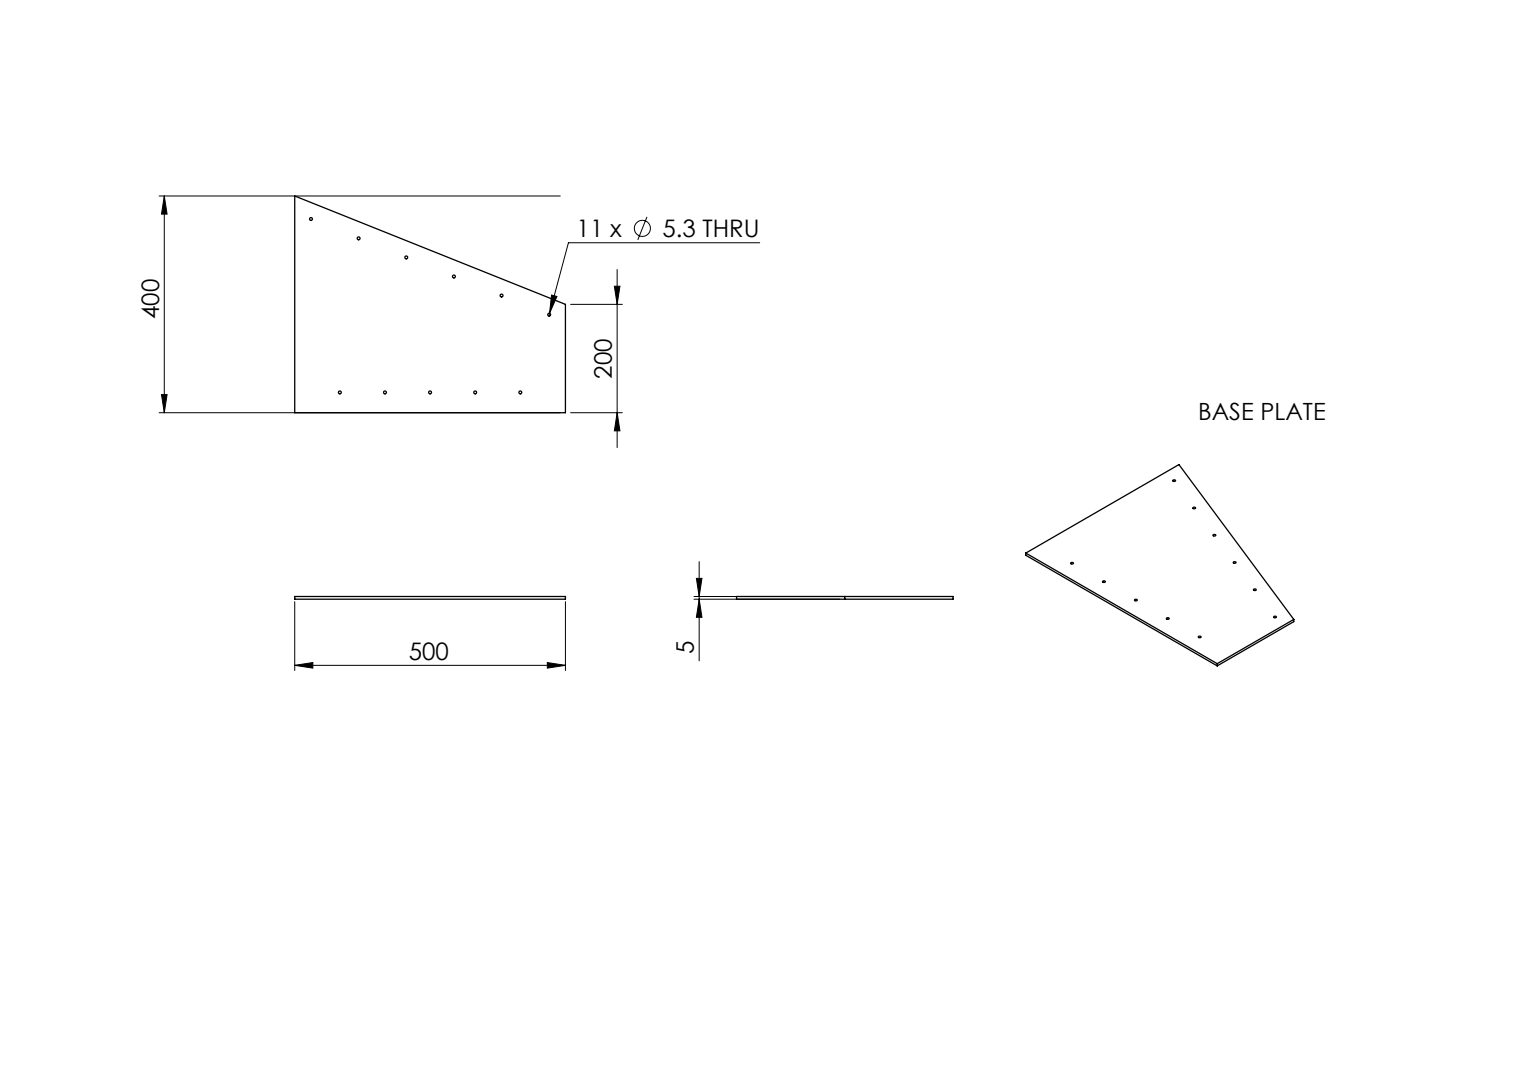
ISO-10303-21;
HEADER;
FILE_DESCRIPTION (('STEP AP214'),
    '1' );
FILE_NAME ('base plate.step',
    '2026-10-24T11:01:53',
    ( '' ),
    ( '' ),
    'SwSTEP 2.0',
    'SolidWorks 2026',
    '' );
FILE_SCHEMA (( 'AUTOMOTIVE_DESIGN' ));
ENDSEC;

DATA;
#2=DIRECTION ( 'NONE',  ( 0.000000000000000000, 0.000000000000000000, 1.000000000000000000 ) ) ;
#30=EDGE_CURVE ( 'NONE', #66, #5441, #6753, .T. ) ;
#34=CIRCLE ( 'NONE', #8257, 2.649999999999985700 ) ;
#39=CARTESIAN_POINT ( 'NONE',  ( 264.0000000000000000, -20.00000000000000000, -48.78142504031547588 ) ) ;
#45=CARTESIAN_POINT ( 'NONE',  ( 352.0000000000000000, -25.00000000000000000, -18.88142504031545243 ) ) ;
#50=DIRECTION ( 'NONE',  ( -0.000000000000000000, 1.000000000000000000, -0.000000000000000000 ) ) ;
#66=VERTEX_POINT ( 'NONE', #8006 ) ;
#72=DIRECTION ( 'NONE',  ( 0.000000000000000000, 0.000000000000000000, 1.000000000000000000 ) ) ;
#74=EDGE_LOOP ( 'NONE', ( #3526, #1411, #5391, #5718 ) ) ;
#79=DIRECTION ( 'NONE',  ( 0.000000000000000000, 0.000000000000000000, 1.000000000000000000 ) ) ;
#80=CIRCLE ( 'NONE', #1767, 2.649999999999985700 ) ;
#95=ORIENTED_EDGE ( 'NONE', *, *, #1233, .T. ) ;
#99=EDGE_LOOP ( 'NONE', ( #6356, #2611 ) ) ;
#101=VERTEX_POINT ( 'NONE', #4083 ) ;
#106=ORIENTED_EDGE ( 'NONE', *, *, #3433, .T. ) ;
#108=CIRCLE ( 'NONE', #2620, 2.649999999999985700 ) ;
#116=LINE ( 'NONE', #6740, #7265 ) ;
#151=CARTESIAN_POINT ( 'NONE',  ( 264.0000000000000000, -20.00000000000000000, -51.43142504031546025 ) ) ;
#152=CARTESIAN_POINT ( 'NONE',  ( 0.000000000000000000, -20.00000000000000000, -154.8500000000000512 ) ) ;
#171=VECTOR ( 'NONE', #2949, 1000.000000000000000 ) ;
#173=VECTOR ( 'NONE', #7716, 1000.000000000000000 ) ;
#196=AXIS2_PLACEMENT_3D ( 'NONE', #7241, #2034, #5327 ) ;
#213=AXIS2_PLACEMENT_3D ( 'NONE', #3905, #5378, #2079 ) ;
#219=CARTESIAN_POINT ( 'NONE',  ( 386.6666666666666288, -20.00000000000000000, 162.5000000000000853 ) ) ;
#228=ORIENTED_EDGE ( 'NONE', *, *, #2374, .T. ) ;
#229=ORIENTED_EDGE ( 'NONE', *, *, #1735, .F. ) ;
#235=EDGE_CURVE ( 'NONE', #6809, #4852, #8223, .T. ) ;
#246=DIRECTION ( 'NONE',  ( 0.000000000000000000, 1.000000000000000000, 0.000000000000000000 ) ) ;
#257=AXIS2_PLACEMENT_3D ( 'NONE', #4957, #2556, #3896 ) ;
#288=EDGE_CURVE ( 'NONE', #3976, #6369, #1904, .T. ) ;
#292=ORIENTED_EDGE ( 'NONE', *, *, #6462, .T. ) ;
#295=EDGE_LOOP ( 'NONE', ( #7507, #2657, #3424, #1885 ) ) ;
#301=AXIS2_PLACEMENT_3D ( 'NONE', #6411, #4498, #8473 ) ;
#359=CIRCLE ( 'NONE', #3284, 2.649999999999985700 ) ;
#372=SURFACE_STYLE_USAGE ( .BOTH. , #1644 ) ;
#376=ORIENTED_EDGE ( 'NONE', *, *, #8589, .T. ) ;
#382=EDGE_LOOP ( 'NONE', ( #940, #229 ) ) ;
#387=LINE ( 'NONE', #1178, #6990 ) ;
#397=ADVANCED_FACE ( 'NONE', ( #5238 ), #7161, .F. ) ;
#402=PLANE ( 'NONE',  #6759 ) ;
#414=DIRECTION ( 'NONE',  ( -0.000000000000000000, 1.000000000000000000, -0.000000000000000000 ) ) ;
#417=CARTESIAN_POINT ( 'NONE',  ( 0.000000000000000000, -20.00000000000000000, -157.5000000000000284 ) ) ;
#424=PRODUCT_DEFINITION ( 'UNKNOWN', '', #7110, #637 ) ;
#437=VERTEX_POINT ( 'NONE', #5072 ) ;
#439=ADVANCED_FACE ( 'NONE', ( #6505 ), #3771, .T. ) ;
#449=VECTOR ( 'NONE', #5880, 1000.000000000000000 ) ;
#452=DIRECTION ( 'NONE',  ( 0.000000000000000000, 0.000000000000000000, 1.000000000000000000 ) ) ;
#453=AXIS2_PLACEMENT_3D ( 'NONE', #5882, #3158, #8554 ) ;
#461=DIRECTION ( 'NONE',  ( 0.000000000000000000, 1.000000000000000000, 0.000000000000000000 ) ) ;
#462=COLOUR_RGB ( '',0.8941176470588234615, 0.8941176470588234615, 0.8941176470588234615 ) ;
#463=ORIENTED_EDGE ( 'NONE', *, *, #2493, .F. ) ;
#464=DIRECTION ( 'NONE',  ( 0.000000000000000000, 0.000000000000000000, 1.000000000000000000 ) ) ;
#469=CIRCLE ( 'NONE', #5320, 2.649999999999985700 ) ;
#487=ORIENTED_EDGE ( 'NONE', *, *, #5222, .T. ) ;
#492=FACE_BOUND ( 'NONE', #3080, .T. ) ;
#499=VECTOR ( 'NONE', #1824, 1000.000000000000000 ) ;
#511=AXIS2_PLACEMENT_3D ( 'NONE', #6789, #836, #2326 ) ;
#523=DIRECTION ( 'NONE',  ( -0.000000000000000000, -0.000000000000000000, -1.000000000000000000 ) ) ;
#532=FACE_BOUND ( 'NONE', #1186, .T. ) ;
#534=DIRECTION ( 'NONE',  ( 0.000000000000000000, 1.000000000000000000, 0.000000000000000000 ) ) ;
#541=CARTESIAN_POINT ( 'NONE',  ( 136.6666666666666288, -20.00000000000000000, 159.8500000000001080 ) ) ;
#542=VERTEX_POINT ( 'NONE', #2423 ) ;
#557=ADVANCED_FACE ( 'NONE', ( #3066, #4491, #7149, #1189, #3755, #5751, #532, #2545, #5707, #1264, #492, #1890 ), #402, .F. ) ;
#558=ORIENTED_EDGE ( 'NONE', *, *, #1197, .T. ) ;
#583=CARTESIAN_POINT ( 'NONE',  ( 219.9999999999999716, -20.00000000000000000, 162.5000000000000853 ) ) ;
#587=AXIS2_PLACEMENT_3D ( 'NONE', #8475, #2553, #2629 ) ;
#590=VERTEX_POINT ( 'NONE', #1227 ) ;
#594=AXIS2_PLACEMENT_3D ( 'NONE', #3123, #464, #5764 ) ;
#602=ORIENTED_EDGE ( 'NONE', *, *, #5769, .F. ) ;
#626=DIRECTION ( 'NONE',  ( 0.000000000000000000, 0.000000000000000000, 1.000000000000000000 ) ) ;
#627=EDGE_CURVE ( 'NONE', #5001, #8500, #3020, .T. ) ;
#635=CARTESIAN_POINT ( 'NONE',  ( 88.00000000000000000, -20.00000000000000000, -121.8314250403154659 ) ) ;
#637=PRODUCT_DEFINITION_CONTEXT ( 'detailed design', #7921, 'design' ) ;
#645=ORIENTED_EDGE ( 'NONE', *, *, #8589, .F. ) ;
#678=VERTEX_POINT ( 'NONE', #39 ) ;
#699=DIRECTION ( 'NONE',  ( 0.000000000000000000, 0.000000000000000000, 1.000000000000000000 ) ) ;
#701=LINE ( 'NONE', #6002, #1786 ) ;
#702=VERTEX_POINT ( 'NONE', #1004 ) ;
#713=ORIENTED_EDGE ( 'NONE', *, *, #3006, .F. ) ;
#723=PLANE ( 'NONE',  #213 ) ;
#742=ADVANCED_FACE ( 'NONE', ( #3927 ), #2016, .F. ) ;
#745=EDGE_CURVE ( 'NONE', #1823, #8068, #1628, .T. ) ;
#769=CARTESIAN_POINT ( 'NONE',  ( 88.00000000000000000, -20.00000000000000000, -119.1814250403154745 ) ) ;
#770=FACE_OUTER_BOUND ( 'NONE', #6133, .T. ) ;
#790=ORIENTED_EDGE ( 'NONE', *, *, #3133, .F. ) ;
#794=EDGE_CURVE ( 'NONE', #7699, #1878, #8026, .T. ) ;
#807=VERTEX_POINT ( 'NONE', #1006 ) ;
#811=EDGE_LOOP ( 'NONE', ( #463, #5711, #6252, #6400 ) ) ;
#818=EDGE_LOOP ( 'NONE', ( #7207, #3911, #376, #7380 ) ) ;
#821=CIRCLE ( 'NONE', #5944, 2.649999999999985700 ) ;
#825=DIRECTION ( 'NONE',  ( -0.000000000000000000, 1.000000000000000000, -0.000000000000000000 ) ) ;
#835=AXIS2_PLACEMENT_3D ( 'NONE', #4055, #2668, #1934 ) ;
#836=DIRECTION ( 'NONE',  ( -0.000000000000000000, 1.000000000000000000, -0.000000000000000000 ) ) ;
#843=DIRECTION ( 'NONE',  ( -0.000000000000000000, -0.000000000000000000, -1.000000000000000000 ) ) ;
#851=EDGE_LOOP ( 'NONE', ( #4373, #2830 ) ) ;
#871=AXIS2_PLACEMENT_3D ( 'NONE', #6654, #7187, #699 ) ;
#873=DIRECTION ( 'NONE',  ( -0.000000000000000000, 1.000000000000000000, -0.000000000000000000 ) ) ;
#875=ORIENTED_EDGE ( 'NONE', *, *, #2374, .F. ) ;
#878=FACE_BOUND ( 'NONE', #2157, .T. ) ;
#912=DIRECTION ( 'NONE',  ( -0.000000000000000000, 1.000000000000000000, -0.000000000000000000 ) ) ;
#921=FACE_BOUND ( 'NONE', #2013, .T. ) ;
#929=AXIS2_PLACEMENT_3D ( 'NONE', #4850, #7548, #4148 ) ;
#937=AXIS2_PLACEMENT_3D ( 'NONE', #5438, #5912, #7446 ) ;
#940=ORIENTED_EDGE ( 'NONE', *, *, #2023, .F. ) ;
#952=EDGE_LOOP ( 'NONE', ( #6894, #7607 ) ) ;
#965=CARTESIAN_POINT ( 'NONE',  ( -30.00000000000002842, -20.00000000000000000, 200.0000000000000000 ) ) ;
#969=ORIENTED_EDGE ( 'NONE', *, *, #7360, .F. ) ;
#995=CARTESIAN_POINT ( 'NONE',  ( 88.00000000000000000, -20.00000000000000000, -121.8314250403154659 ) ) ;
#996=DIRECTION ( 'NONE',  ( 0.000000000000000000, 1.000000000000000000, 0.000000000000000000 ) ) ;
#997=VERTEX_POINT ( 'NONE', #1752 ) ;
#1000=ORIENTED_EDGE ( 'NONE', *, *, #1573, .F. ) ;
#1004=CARTESIAN_POINT ( 'NONE',  ( 0.000000000000000000, -25.00000000000000000, -154.8500000000000512 ) ) ;
#1006=CARTESIAN_POINT ( 'NONE',  ( 264.0000000000000000, -20.00000000000000000, -54.08142504031544462 ) ) ;
#1019=VECTOR ( 'NONE', #8238, 1000.000000000000000 ) ;
#1031=EDGE_LOOP ( 'NONE', ( #8342, #5767, #3173, #2916 ) ) ;
#1058=ADVANCED_FACE ( 'NONE', ( #8581 ), #3438, .F. ) ;
#1060=CARTESIAN_POINT ( 'NONE',  ( 470.0000000000000000, -20.00000000000000000, 200.0000000000000000 ) ) ;
#1077=VERTEX_POINT ( 'NONE', #6603 ) ;
#1100=ORIENTED_EDGE ( 'NONE', *, *, #2407, .F. ) ;
#1112=DIRECTION ( 'NONE',  ( 0.000000000000000000, 0.000000000000000000, 1.000000000000000000 ) ) ;
#1124=CARTESIAN_POINT ( 'NONE',  ( 219.9999999999999716, -20.00000000000000000, 159.8500000000001080 ) ) ;
#1132=ORIENTED_EDGE ( 'NONE', *, *, #1493, .F. ) ;
#1134=LINE ( 'NONE', #5133, #3405 ) ;
#1160=VERTEX_POINT ( 'NONE', #4912 ) ;
#1168=EDGE_CURVE ( 'NONE', #8068, #1823, #2321, .T. ) ;
#1169=ADVANCED_FACE ( 'NONE', ( #2314 ), #6779, .F. ) ;
#1171=ORIENTED_EDGE ( 'NONE', *, *, #5798, .F. ) ;
#1174=CARTESIAN_POINT ( 'NONE',  ( 219.9999999999999716, -20.00000000000000000, 162.5000000000000853 ) ) ;
#1178=CARTESIAN_POINT ( 'NONE',  ( 219.9999999999999716, -20.00000000000000000, 165.1500000000000625 ) ) ;
#1186=EDGE_LOOP ( 'NONE', ( #3554, #4363 ) ) ;
#1189=FACE_BOUND ( 'NONE', #5501, .T. ) ;
#1190=DIRECTION ( 'NONE',  ( 0.000000000000000000, 0.000000000000000000, 1.000000000000000000 ) ) ;
#1197=EDGE_CURVE ( 'NONE', #4852, #5678, #6117, .T. ) ;
#1202=CYLINDRICAL_SURFACE ( 'NONE', #4532, 2.649999999999985700 ) ;
#1207=LINE ( 'NONE', #3864, #3823 ) ;
#1219=CARTESIAN_POINT ( 'NONE',  ( 88.00000000000000000, -25.00000000000000000, -119.1814250403154745 ) ) ;
#1226=EDGE_CURVE ( 'NONE', #702, #8500, #2952, .T. ) ;
#1227=CARTESIAN_POINT ( 'NONE',  ( 303.3333333333333144, -20.00000000000000000, 165.1500000000000625 ) ) ;
#1233=EDGE_CURVE ( 'NONE', #5259, #66, #3566, .T. ) ;
#1264=FACE_BOUND ( 'NONE', #2961, .T. ) ;
#1283=ORIENTED_EDGE ( 'NONE', *, *, #5388, .F. ) ;
#1285=AXIS2_PLACEMENT_3D ( 'NONE', #7939, #6622, #1975 ) ;
#1292=CARTESIAN_POINT ( 'NONE',  ( 219.9999999999999716, -20.00000000000000000, 162.5000000000000853 ) ) ;
#1311=LINE ( 'NONE', #7982, #7625 ) ;
#1325=EDGE_LOOP ( 'NONE', ( #7906, #6774 ) ) ;
#1336=ORIENTED_EDGE ( 'NONE', *, *, #1493, .T. ) ;
#1339=AXIS2_PLACEMENT_3D ( 'NONE', #5714, #7733, #452 ) ;
#1344=AXIS2_PLACEMENT_3D ( 'NONE', #2621, #6085, #6001 ) ;
#1346=CARTESIAN_POINT ( 'NONE',  ( 352.0000000000000000, -20.00000000000000000, -16.23142504031546807 ) ) ;
#1364=CIRCLE ( 'NONE', #3460, 2.649999999999985700 ) ;
#1369=UNCERTAINTY_MEASURE_WITH_UNIT (LENGTH_MEASURE( 1.000000000000000082E-05 ), #4293, 'distance_accuracy_value', 'NONE');
#1370=ORIENTED_EDGE ( 'NONE', *, *, #1684, .T. ) ;
#1371=DIRECTION ( 'NONE',  ( 0.000000000000000000, 0.000000000000000000, 1.000000000000000000 ) ) ;
#1376=EDGE_LOOP ( 'NONE', ( #713, #2858, #5114, #8177 ) ) ;
#1385=ORIENTED_EDGE ( 'NONE', *, *, #1994, .T. ) ;
#1388=CARTESIAN_POINT ( 'NONE',  ( 352.0000000000000000, -25.00000000000000000, -13.58142504031548192 ) ) ;
#1404=CARTESIAN_POINT ( 'NONE',  ( 352.0000000000000000, -20.00000000000000000, -16.23142504031546807 ) ) ;
#1409=EDGE_LOOP ( 'NONE', ( #2213, #1591 ) ) ;
#1411=ORIENTED_EDGE ( 'NONE', *, *, #8314, .T. ) ;
#1412=EDGE_LOOP ( 'NONE', ( #1000, #1132, #7088, #5511 ) ) ;
#1429=ADVANCED_FACE ( 'NONE', ( #8407 ), #2446, .F. ) ;
#1431=DIRECTION ( 'NONE',  ( -0.000000000000000000, 1.000000000000000000, -0.000000000000000000 ) ) ;
#1450=FACE_OUTER_BOUND ( 'NONE', #2004, .T. ) ;
#1451=CARTESIAN_POINT ( 'NONE',  ( 136.6666666666666288, -20.00000000000000000, 165.1500000000000625 ) ) ;
#1458=CARTESIAN_POINT ( 'NONE',  ( 439.9999999999999432, -20.00000000000000000, 18.96857495968446017 ) ) ;
#1462=CARTESIAN_POINT ( 'NONE',  ( 53.33333333333330017, -25.00000000000000000, 165.1500000000000625 ) ) ;
#1469=LINE ( 'NONE', #8144, #2419 ) ;
#1471=AXIS2_PLACEMENT_3D ( 'NONE', #2548, #5905, #72 ) ;
#1493=EDGE_CURVE ( 'NONE', #1660, #542, #6479, .T. ) ;
#1499=DIRECTION ( 'NONE',  ( 0.000000000000000000, 1.000000000000000000, 0.000000000000000000 ) ) ;
#1512=PRODUCT_CONTEXT ( 'NONE', #2313, 'mechanical' ) ;
#1528=DIRECTION ( 'NONE',  ( 0.000000000000000000, -0.000000000000000000, 1.000000000000000000 ) ) ;
#1540=CARTESIAN_POINT ( 'NONE',  ( 53.33333333333330017, -20.00000000000000000, 159.8500000000001080 ) ) ;
#1570=ADVANCED_FACE ( 'NONE', ( #6676 ), #723, .F. ) ;
#1573=EDGE_CURVE ( 'NONE', #542, #807, #4727, .T. ) ;
#1577=VECTOR ( 'NONE', #6770, 1000.000000000000000 ) ;
#1591=ORIENTED_EDGE ( 'NONE', *, *, #7360, .T. ) ;
#1593=EDGE_CURVE ( 'NONE', #4392, #5678, #6106, .T. ) ;
#1609=VERTEX_POINT ( 'NONE', #7426 ) ;
#1611=VERTEX_POINT ( 'NONE', #1462 ) ;
#1616=VECTOR ( 'NONE', #2248, 1000.000000000000000 ) ;
#1620=DIRECTION ( 'NONE',  ( -0.000000000000000000, 1.000000000000000000, -0.000000000000000000 ) ) ;
#1628=CIRCLE ( 'NONE', #2739, 2.649999999999985700 ) ;
#1644=SURFACE_SIDE_STYLE ('',( #3727 ) ) ;
#1655=CARTESIAN_POINT ( 'NONE',  ( 386.6666666666666288, -20.00000000000000000, 165.1500000000000625 ) ) ;
#1660=VERTEX_POINT ( 'NONE', #7562 ) ;
#1663=DIRECTION ( 'NONE',  ( -0.000000000000000000, 1.000000000000000000, -0.000000000000000000 ) ) ;
#1684=EDGE_CURVE ( 'NONE', #4319, #6518, #3553, .T. ) ;
#1688=FILL_AREA_STYLE_COLOUR ( '', #462 ) ;
#1705=DIRECTION ( 'NONE',  ( 0.000000000000000000, 1.000000000000000000, 0.000000000000000000 ) ) ;
#1717=CARTESIAN_POINT ( 'NONE',  ( 136.6666666666666288, -25.00000000000000000, 159.8500000000001080 ) ) ;
#1718=DIRECTION ( 'NONE',  ( 0.000000000000000000, 0.000000000000000000, 1.000000000000000000 ) ) ;
#1729=ORIENTED_EDGE ( 'NONE', *, *, #5789, .F. ) ;
#1735=EDGE_CURVE ( 'NONE', #807, #678, #3279, .T. ) ;
#1746=DIRECTION ( 'NONE',  ( 0.000000000000000000, 0.000000000000000000, 1.000000000000000000 ) ) ;
#1752=CARTESIAN_POINT ( 'NONE',  ( 176.0000000000000000, -20.00000000000000000, -89.28142504031545457 ) ) ;
#1762=EDGE_CURVE ( 'NONE', #590, #7349, #1901, .T. ) ;
#1763=LINE ( 'NONE', #5831, #5405 ) ;
#1767=AXIS2_PLACEMENT_3D ( 'NONE', #1903, #1499, #2763 ) ;
#1775=ORIENTED_EDGE ( 'NONE', *, *, #7658, .T. ) ;
#1776=CARTESIAN_POINT ( 'NONE',  ( 53.33333333333330017, -20.00000000000000000, 165.1500000000000625 ) ) ;
#1782=VERTEX_POINT ( 'NONE', #7778 ) ;
#1786=VECTOR ( 'NONE', #3275, 1000.000000000000000 ) ;
#1792=FACE_OUTER_BOUND ( 'NONE', #4027, .T. ) ;
#1795=DIRECTION ( 'NONE',  ( 0.000000000000000000, 0.000000000000000000, 1.000000000000000000 ) ) ;
#1803=AXIS2_PLACEMENT_3D ( 'NONE', #4582, #6538, #8361 ) ;
#1823=VERTEX_POINT ( 'NONE', #1776 ) ;
#1824=DIRECTION ( 'NONE',  ( -0.000000000000000000, 1.000000000000000000, -0.000000000000000000 ) ) ;
#1833=LINE ( 'NONE', #3007, #173 ) ;
#1839=EDGE_CURVE ( 'NONE', #702, #1160, #359, .T. ) ;
#1844=EDGE_CURVE ( 'NONE', #7459, #1077, #3980, .T. ) ;
#1864=ADVANCED_FACE ( 'NONE', ( #4026 ), #1202, .F. ) ;
#1866=ORIENTED_EDGE ( 'NONE', *, *, #2769, .F. ) ;
#1869=CIRCLE ( 'NONE', #6709, 2.649999999999985700 ) ;
#1878=VERTEX_POINT ( 'NONE', #541 ) ;
#1884=DIRECTION ( 'NONE',  ( 0.000000000000000000, 1.000000000000000000, 0.000000000000000000 ) ) ;
#1885=ORIENTED_EDGE ( 'NONE', *, *, #794, .T. ) ;
#1890=FACE_OUTER_BOUND ( 'NONE', #7744, .T. ) ;
#1901=CIRCLE ( 'NONE', #4663, 2.649999999999985700 ) ;
#1903=CARTESIAN_POINT ( 'NONE',  ( 439.9999999999999432, -25.00000000000000000, 18.96857495968446017 ) ) ;
#1904=CIRCLE ( 'NONE', #2038, 2.649999999999985700 ) ;
#1909=CARTESIAN_POINT ( 'NONE',  ( 352.0000000000000000, -20.00000000000000000, -18.88142504031545243 ) ) ;
#1931=EDGE_CURVE ( 'NONE', #2500, #5031, #8160, .T. ) ;
#1934=DIRECTION ( 'NONE',  ( 0.000000000000000000, 0.000000000000000000, 1.000000000000000000 ) ) ;
#1947=CYLINDRICAL_SURFACE ( 'NONE', #6109, 2.649999999999985700 ) ;
#1961=CARTESIAN_POINT ( 'NONE',  ( -30.00000000000002842, -20.00000000000000000, -200.0000000000000000 ) ) ;
#1965=DIRECTION ( 'NONE',  ( -0.000000000000000000, 1.000000000000000000, -0.000000000000000000 ) ) ;
#1975=DIRECTION ( 'NONE',  ( 0.000000000000000000, 0.000000000000000000, 1.000000000000000000 ) ) ;
#1982=DIRECTION ( 'NONE',  ( 0.000000000000000000, 0.000000000000000000, 1.000000000000000000 ) ) ;
#1983=ORIENTED_EDGE ( 'NONE', *, *, #5161, .T. ) ;
#1987=AXIS2_PLACEMENT_3D ( 'NONE', #5470, #3435, #4736 ) ;
#1989=AXIS2_PLACEMENT_3D ( 'NONE', #5997, #3404, #5221 ) ;
#1994=EDGE_CURVE ( 'NONE', #2349, #6072, #80, .T. ) ;
#2004=EDGE_LOOP ( 'NONE', ( #4240, #6741, #4572, #4137 ) ) ;
#2013=EDGE_LOOP ( 'NONE', ( #7119, #1866 ) ) ;
#2016=CYLINDRICAL_SURFACE ( 'NONE', #1344, 2.649999999999985700 ) ;
#2021=FACE_BOUND ( 'NONE', #952, .T. ) ;
#2023=EDGE_CURVE ( 'NONE', #678, #807, #6612, .T. ) ;
#2034=DIRECTION ( 'NONE',  ( -0.000000000000000000, 1.000000000000000000, -0.000000000000000000 ) ) ;
#2038=AXIS2_PLACEMENT_3D ( 'NONE', #4251, #6901, #4860 ) ;
#2054=VECTOR ( 'NONE', #7575, 1000.000000000000000 ) ;
#2065=CYLINDRICAL_SURFACE ( 'NONE', #835, 2.649999999999985700 ) ;
#2076=DIRECTION ( 'NONE',  ( 0.000000000000000000, 0.000000000000000000, 1.000000000000000000 ) ) ;
#2079=DIRECTION ( 'NONE',  ( -1.000000000000000000, 0.000000000000000000, -0.000000000000000000 ) ) ;
#2090=LINE ( 'NONE', #2593, #5948 ) ;
#2102=DIRECTION ( 'NONE',  ( -0.000000000000000000, 1.000000000000000000, -0.000000000000000000 ) ) ;
#2111=CARTESIAN_POINT ( 'NONE',  ( 176.0000000000000000, -25.00000000000000000, -89.28142504031545457 ) ) ;
#2112=EDGE_CURVE ( 'NONE', #7579, #6119, #5229, .T. ) ;
#2119=CARTESIAN_POINT ( 'NONE',  ( 53.33333333333330017, -20.00000000000000000, 165.1500000000000625 ) ) ;
#2124=CARTESIAN_POINT ( 'NONE',  ( 386.6666666666666288, -25.00000000000000000, 162.5000000000000853 ) ) ;
#2151=FACE_OUTER_BOUND ( 'NONE', #818, .T. ) ;
#2157=EDGE_LOOP ( 'NONE', ( #4864, #7382 ) ) ;
#2196=MECHANICAL_DESIGN_GEOMETRIC_PRESENTATION_REPRESENTATION('',(#6917),#5930);
#2204=ORIENTED_EDGE ( 'NONE', *, *, #6722, .T. ) ;
#2212=ORIENTED_EDGE ( 'NONE', *, *, #1197, .F. ) ;
#2213=ORIENTED_EDGE ( 'NONE', *, *, #5279, .T. ) ;
#2236=DIRECTION ( 'NONE',  ( 0.000000000000000000, 0.000000000000000000, 1.000000000000000000 ) ) ;
#2242=ORIENTED_EDGE ( 'NONE', *, *, #6880, .T. ) ;
#2245=DIRECTION ( 'NONE',  ( -0.000000000000000000, 1.000000000000000000, -0.000000000000000000 ) ) ;
#2248=DIRECTION ( 'NONE',  ( -0.000000000000000000, -0.000000000000000000, -1.000000000000000000 ) ) ;
#2263=MANIFOLD_SOLID_BREP ( 'Cut-Extrude1', #4113 ) ;
#2276=FACE_BOUND ( 'NONE', #851, .T. ) ;
#2282=ORIENTED_EDGE ( 'NONE', *, *, #4122, .T. ) ;
#2304=CARTESIAN_POINT ( 'NONE',  ( 470.0000000000000000, -20.00000000000000000, 200.0000000000000000 ) ) ;
#2306=CARTESIAN_POINT ( 'NONE',  ( 107.9310344827585908, -25.00000000000000000, -144.8275862068965125 ) ) ;
#2310=CARTESIAN_POINT ( 'NONE',  ( 176.0000000000000000, -20.00000000000000000, -83.98142504031548583 ) ) ;
#2313=APPLICATION_CONTEXT ( 'automotive_design' ) ;
#2314=FACE_OUTER_BOUND ( 'NONE', #3354, .T. ) ;
#2321=CIRCLE ( 'NONE', #5352, 2.649999999999985700 ) ;
#2323=FACE_OUTER_BOUND ( 'NONE', #4142, .T. ) ;
#2326=DIRECTION ( 'NONE',  ( 0.000000000000000000, 0.000000000000000000, 1.000000000000000000 ) ) ;
#2336=CARTESIAN_POINT ( 'NONE',  ( -30.00000000000002842, -25.00000000000000000, 200.0000000000000000 ) ) ;
#2343=DIRECTION ( 'NONE',  ( -0.000000000000000000, 1.000000000000000000, -0.000000000000000000 ) ) ;
#2347=CARTESIAN_POINT ( 'NONE',  ( 0.000000000000000000, -25.00000000000000000, -157.5000000000000284 ) ) ;
#2349=VERTEX_POINT ( 'NONE', #3236 ) ;
#2357=CARTESIAN_POINT ( 'NONE',  ( 352.0000000000000000, -25.00000000000000000, -16.23142504031546807 ) ) ;
#2374=EDGE_CURVE ( 'NONE', #6072, #3976, #1311, .T. ) ;
#2384=ORIENTED_EDGE ( 'NONE', *, *, #6116, .F. ) ;
#2407=EDGE_CURVE ( 'NONE', #101, #6809, #701, .T. ) ;
#2419=VECTOR ( 'NONE', #7477, 1000.000000000000000 ) ;
#2423=CARTESIAN_POINT ( 'NONE',  ( 264.0000000000000000, -25.00000000000000000, -54.08142504031544462 ) ) ;
#2446=CYLINDRICAL_SURFACE ( 'NONE', #5223, 2.649999999999985700 ) ;
#2447=EDGE_LOOP ( 'NONE', ( #4684, #602, #95, #7172 ) ) ;
#2449=CARTESIAN_POINT ( 'NONE',  ( 303.3333333333333144, -20.00000000000000000, 162.5000000000000853 ) ) ;
#2463=VECTOR ( 'NONE', #7868, 1000.000000000000000 ) ;
#2470=AXIS2_PLACEMENT_3D ( 'NONE', #5762, #6331, #3162 ) ;
#2484=DIRECTION ( 'NONE',  ( 0.000000000000000000, 1.000000000000000000, 0.000000000000000000 ) ) ;
#2493=EDGE_CURVE ( 'NONE', #1782, #7349, #2839, .T. ) ;
#2500=VERTEX_POINT ( 'NONE', #8156 ) ;
#2506=DIRECTION ( 'NONE',  ( 0.000000000000000000, -0.000000000000000000, 1.000000000000000000 ) ) ;
#2514=VECTOR ( 'NONE', #2846, 1000.000000000000000 ) ;
#2516=ORIENTED_EDGE ( 'NONE', *, *, #5862, .T. ) ;
#2523=ORIENTED_EDGE ( 'NONE', *, *, #3038, .T. ) ;
#2529=ORIENTED_EDGE ( 'NONE', *, *, #8506, .T. ) ;
#2545=FACE_BOUND ( 'NONE', #1409, .T. ) ;
#2548=CARTESIAN_POINT ( 'NONE',  ( 0.000000000000000000, -20.00000000000000000, -157.5000000000000284 ) ) ;
#2553=DIRECTION ( 'NONE',  ( 0.000000000000000000, 1.000000000000000000, 0.000000000000000000 ) ) ;
#2556=DIRECTION ( 'NONE',  ( 0.000000000000000000, 1.000000000000000000, 0.000000000000000000 ) ) ;
#2567=CARTESIAN_POINT ( 'NONE',  ( 264.0000000000000000, -20.00000000000000000, -54.08142504031544462 ) ) ;
#2580=EDGE_LOOP ( 'NONE', ( #5590, #6632, #2724, #1983 ) ) ;
#2587=EDGE_CURVE ( 'NONE', #1160, #5001, #4181, .T. ) ;
#2593=CARTESIAN_POINT ( 'NONE',  ( 176.0000000000000000, -20.00000000000000000, -89.28142504031545457 ) ) ;
#2611=ORIENTED_EDGE ( 'NONE', *, *, #627, .F. ) ;
#2620=AXIS2_PLACEMENT_3D ( 'NONE', #7882, #1884, #7263 ) ;
#2621=CARTESIAN_POINT ( 'NONE',  ( 53.33333333333330017, -20.00000000000000000, 162.5000000000000853 ) ) ;
#2629=DIRECTION ( 'NONE',  ( 0.000000000000000000, 0.000000000000000000, 1.000000000000000000 ) ) ;
#2640=DIRECTION ( 'NONE',  ( 0.000000000000000000, 0.000000000000000000, 1.000000000000000000 ) ) ;
#2657=ORIENTED_EDGE ( 'NONE', *, *, #3036, .F. ) ;
#2660=ADVANCED_FACE ( 'NONE', ( #7721 ), #5137, .F. ) ;
#2668=DIRECTION ( 'NONE',  ( -0.000000000000000000, 1.000000000000000000, -0.000000000000000000 ) ) ;
#2707=SHAPE_REPRESENTATION ( 'base plate', ( #594 ), #6566 ) ;
#2709=CARTESIAN_POINT ( 'NONE',  ( 88.00000000000000000, -25.00000000000000000, -121.8314250403154659 ) ) ;
#2716=FACE_OUTER_BOUND ( 'NONE', #2447, .T. ) ;
#2719=CARTESIAN_POINT ( 'NONE',  ( 303.3333333333333144, -20.00000000000000000, 162.5000000000000853 ) ) ;
#2724=ORIENTED_EDGE ( 'NONE', *, *, #1226, .T. ) ;
#2725=EDGE_LOOP ( 'NONE', ( #3417, #3665, #3898, #6958 ) ) ;
#2739=AXIS2_PLACEMENT_3D ( 'NONE', #6572, #3274, #5263 ) ;
#2742=EDGE_CURVE ( 'NONE', #6803, #7313, #108, .T. ) ;
#2759=LINE ( 'NONE', #6006, #449 ) ;
#2760=CARTESIAN_POINT ( 'NONE',  ( 470.0000000000000000, -25.00000000000000000, 200.0000000000000000 ) ) ;
#2763=DIRECTION ( 'NONE',  ( 0.000000000000000000, 0.000000000000000000, 1.000000000000000000 ) ) ;
#2764=VECTOR ( 'NONE', #1620, 1000.000000000000000 ) ;
#2769=EDGE_CURVE ( 'NONE', #5441, #66, #7484, .T. ) ;
#2802=VECTOR ( 'NONE', #3586, 1000.000000000000000 ) ;
#2810=EDGE_CURVE ( 'NONE', #1077, #7459, #1364, .T. ) ;
#2825=CIRCLE ( 'NONE', #1987, 2.649999999999985700 ) ;
#2829=EDGE_CURVE ( 'NONE', #8049, #997, #821, .T. ) ;
#2830=ORIENTED_EDGE ( 'NONE', *, *, #4495, .F. ) ;
#2836=FACE_BOUND ( 'NONE', #3650, .T. ) ;
#2839=LINE ( 'NONE', #4927, #8336 ) ;
#2846=DIRECTION ( 'NONE',  ( -0.000000000000000000, 1.000000000000000000, -0.000000000000000000 ) ) ;
#2858=ORIENTED_EDGE ( 'NONE', *, *, #3577, .F. ) ;
#2864=ORIENTED_EDGE ( 'NONE', *, *, #5439, .F. ) ;
#2887=LINE ( 'NONE', #6970, #2514 ) ;
#2914=CYLINDRICAL_SURFACE ( 'NONE', #3100, 2.649999999999985700 ) ;
#2916=ORIENTED_EDGE ( 'NONE', *, *, #1226, .F. ) ;
#2942=( NAMED_UNIT ( * ) PLANE_ANGLE_UNIT ( ) SI_UNIT ( $, .RADIAN. ) );
#2949=DIRECTION ( 'NONE',  ( -0.000000000000000000, 1.000000000000000000, -0.000000000000000000 ) ) ;
#2950=FACE_OUTER_BOUND ( 'NONE', #1412, .T. ) ;
#2952=LINE ( 'NONE', #152, #7867 ) ;
#2956=ORIENTED_EDGE ( 'NONE', *, *, #7731, .F. ) ;
#2961=EDGE_LOOP ( 'NONE', ( #7824, #6467 ) ) ;
#2964=CARTESIAN_POINT ( 'NONE',  ( 352.0000000000000000, -20.00000000000000000, -13.58142504031548192 ) ) ;
#2966=AXIS2_PLACEMENT_3D ( 'NONE', #5977, #7951, #7242 ) ;
#2973=DIRECTION ( 'NONE',  ( -0.000000000000000000, 1.000000000000000000, -0.000000000000000000 ) ) ;
#3004=ORIENTED_EDGE ( 'NONE', *, *, #7979, .F. ) ;
#3005=VECTOR ( 'NONE', #246, 1000.000000000000000 ) ;
#3006=EDGE_CURVE ( 'NONE', #7579, #997, #2090, .T. ) ;
#3007=CARTESIAN_POINT ( 'NONE',  ( 88.00000000000000000, -20.00000000000000000, -124.4814250403154574 ) ) ;
#3020=CIRCLE ( 'NONE', #937, 2.649999999999985700 ) ;
#3026=ORIENTED_EDGE ( 'NONE', *, *, #2112, .F. ) ;
#3031=DIRECTION ( 'NONE',  ( -0.000000000000000000, 1.000000000000000000, -0.000000000000000000 ) ) ;
#3036=EDGE_CURVE ( 'NONE', #5928, #5141, #4019, .T. ) ;
#3038=EDGE_CURVE ( 'NONE', #7972, #6999, #3885, .T. ) ;
#3039=PRESENTATION_STYLE_ASSIGNMENT (( #372 ) ) ;
#3044=CARTESIAN_POINT ( 'NONE',  ( 136.6666666666666288, -25.00000000000000000, 165.1500000000000625 ) ) ;
#3054=CYLINDRICAL_SURFACE ( 'NONE', #5049, 2.649999999999985700 ) ;
#3066=FACE_BOUND ( 'NONE', #3636, .T. ) ;
#3080=EDGE_LOOP ( 'NONE', ( #487, #7113 ) ) ;
#3090=EDGE_LOOP ( 'NONE', ( #4873, #3990, #5523, #8304 ) ) ;
#3100=AXIS2_PLACEMENT_3D ( 'NONE', #4175, #873, #3528 ) ;
#3123=CARTESIAN_POINT ( 'NONE',  ( 0.000000000000000000, 0.000000000000000000, 0.000000000000000000 ) ) ;
#3133=EDGE_CURVE ( 'NONE', #3710, #1611, #3324, .T. ) ;
#3158=DIRECTION ( 'NONE',  ( 0.000000000000000000, 1.000000000000000000, 0.000000000000000000 ) ) ;
#3162=DIRECTION ( 'NONE',  ( 0.000000000000000000, 0.000000000000000000, 1.000000000000000000 ) ) ;
#3173=ORIENTED_EDGE ( 'NONE', *, *, #627, .T. ) ;
#3179=FACE_OUTER_BOUND ( 'NONE', #1376, .T. ) ;
#3195=DIRECTION ( 'NONE',  ( 0.000000000000000000, 0.000000000000000000, 1.000000000000000000 ) ) ;
#3207=DIRECTION ( 'NONE',  ( -0.000000000000000000, 0.000000000000000000, -1.000000000000000000 ) ) ;
#3210=DIRECTION ( 'NONE',  ( 0.3713906763541037215, 0.000000000000000000, -0.9284766908852594147 ) ) ;
#3227=ORIENTED_EDGE ( 'NONE', *, *, #6043, .T. ) ;
#3236=CARTESIAN_POINT ( 'NONE',  ( 439.9999999999999432, -25.00000000000000000, 16.31857495968447225 ) ) ;
#3239=EDGE_CURVE ( 'NONE', #5928, #7699, #4760, .T. ) ;
#3274=DIRECTION ( 'NONE',  ( -0.000000000000000000, 1.000000000000000000, -0.000000000000000000 ) ) ;
#3275=DIRECTION ( 'NONE',  ( 0.000000000000000000, -1.000000000000000000, 0.000000000000000000 ) ) ;
#3279=CIRCLE ( 'NONE', #4526, 2.649999999999985700 ) ;
#3284=AXIS2_PLACEMENT_3D ( 'NONE', #2347, #461, #3634 ) ;
#3291=DIRECTION ( 'NONE',  ( -0.000000000000000000, 1.000000000000000000, -0.000000000000000000 ) ) ;
#3303=ORIENTED_EDGE ( 'NONE', *, *, #7658, .F. ) ;
#3310=CARTESIAN_POINT ( 'NONE',  ( 386.6666666666666288, -20.00000000000000000, 162.5000000000000853 ) ) ;
#3319=ORIENTED_EDGE ( 'NONE', *, *, #2810, .T. ) ;
#3324=CIRCLE ( 'NONE', #257, 2.649999999999985700 ) ;
#3345=DIRECTION ( 'NONE',  ( 0.000000000000000000, 0.000000000000000000, 1.000000000000000000 ) ) ;
#3354=EDGE_LOOP ( 'NONE', ( #2864, #4104, #5130, #6098 ) ) ;
#3360=EDGE_LOOP ( 'NONE', ( #1171, #2956, #2204, #3319 ) ) ;
#3364=CARTESIAN_POINT ( 'NONE',  ( 264.0000000000000000, -20.00000000000000000, -51.43142504031546025 ) ) ;
#3366=AXIS2_PLACEMENT_3D ( 'NONE', #4799, #7453, #5492 ) ;
#3367=DIRECTION ( 'NONE',  ( -0.000000000000000000, 1.000000000000000000, -0.000000000000000000 ) ) ;
#3404=DIRECTION ( 'NONE',  ( 0.000000000000000000, 1.000000000000000000, 0.000000000000000000 ) ) ;
#3405=VECTOR ( 'NONE', #523, 1000.000000000000000 ) ;
#3417=ORIENTED_EDGE ( 'NONE', *, *, #5495, .F. ) ;
#3424=ORIENTED_EDGE ( 'NONE', *, *, #3239, .T. ) ;
#3433=EDGE_CURVE ( 'NONE', #4319, #101, #1763, .T. ) ;
#3434=ORIENTED_EDGE ( 'NONE', *, *, #7897, .T. ) ;
#3435=DIRECTION ( 'NONE',  ( 0.000000000000000000, 1.000000000000000000, 0.000000000000000000 ) ) ;
#3438=CYLINDRICAL_SURFACE ( 'NONE', #1471, 2.649999999999985700 ) ;
#3460=AXIS2_PLACEMENT_3D ( 'NONE', #1346, #5906, #5216 ) ;
#3503=EDGE_LOOP ( 'NONE', ( #7128, #6767, #6332, #7667 ) ) ;
#3526=ORIENTED_EDGE ( 'NONE', *, *, #7820, .F. ) ;
#3528=DIRECTION ( 'NONE',  ( 0.000000000000000000, 0.000000000000000000, 1.000000000000000000 ) ) ;
#3532=AXIS2_PLACEMENT_3D ( 'NONE', #6197, #2245, #1371 ) ;
#3539=VECTOR ( 'NONE', #3616, 1000.000000000000000 ) ;
#3549=CYLINDRICAL_SURFACE ( 'NONE', #3532, 2.649999999999985700 ) ;
#3553=LINE ( 'NONE', #2304, #7311 ) ;
#3554=ORIENTED_EDGE ( 'NONE', *, *, #5769, .T. ) ;
#3566=LINE ( 'NONE', #1655, #2054 ) ;
#3568=ORIENTED_EDGE ( 'NONE', *, *, #4284, .T. ) ;
#3577=EDGE_CURVE ( 'NONE', #6119, #7579, #7650, .T. ) ;
#3582=CARTESIAN_POINT ( 'NONE',  ( 88.00000000000000000, -20.00000000000000000, -119.1814250403154745 ) ) ;
#3583=DIRECTION ( 'NONE',  ( -0.000000000000000000, 1.000000000000000000, -0.000000000000000000 ) ) ;
#3586=DIRECTION ( 'NONE',  ( 0.000000000000000000, 1.000000000000000000, 0.000000000000000000 ) ) ;
#3616=DIRECTION ( 'NONE',  ( 1.000000000000000000, 0.000000000000000000, 0.000000000000000000 ) ) ;
#3622=CYLINDRICAL_SURFACE ( 'NONE', #7968, 2.649999999999985700 ) ;
#3627=ORIENTED_EDGE ( 'NONE', *, *, #7979, .T. ) ;
#3630=CARTESIAN_POINT ( 'NONE',  ( 352.0000000000000000, -25.00000000000000000, -16.23142504031546807 ) ) ;
#3634=DIRECTION ( 'NONE',  ( 0.000000000000000000, 0.000000000000000000, 1.000000000000000000 ) ) ;
#3636=EDGE_LOOP ( 'NONE', ( #3568, #1385 ) ) ;
#3637=FILL_AREA_STYLE ('',( #1688 ) ) ;
#3650=EDGE_LOOP ( 'NONE', ( #4542, #4088 ) ) ;
#3658=AXIS2_PLACEMENT_3D ( 'NONE', #2124, #6073, #7521 ) ;
#3660=ADVANCED_FACE ( 'NONE', ( #2716 ), #2065, .F. ) ;
#3665=ORIENTED_EDGE ( 'NONE', *, *, #1573, .T. ) ;
#3686=EDGE_LOOP ( 'NONE', ( #8514, #4305, #7468, #875 ) ) ;
#3707=DIRECTION ( 'NONE',  ( -0.000000000000000000, 1.000000000000000000, -0.000000000000000000 ) ) ;
#3710=VERTEX_POINT ( 'NONE', #5916 ) ;
#3723=DIRECTION ( 'NONE',  ( 0.000000000000000000, 0.000000000000000000, 1.000000000000000000 ) ) ;
#3726=EDGE_LOOP ( 'NONE', ( #6175, #2523 ) ) ;
#3727=SURFACE_STYLE_FILL_AREA ( #3637 ) ;
#3755=FACE_BOUND ( 'NONE', #4605, .T. ) ;
#3756=AXIS2_PLACEMENT_3D ( 'NONE', #5776, #6305, #1746 ) ;
#3768=DIRECTION ( 'NONE',  ( -0.000000000000000000, 1.000000000000000000, -0.000000000000000000 ) ) ;
#3771=PLANE ( 'NONE',  #6486 ) ;
#3812=DIRECTION ( 'NONE',  ( 0.000000000000000000, 0.000000000000000000, 1.000000000000000000 ) ) ;
#3823=VECTOR ( 'NONE', #5932, 1000.000000000000114 ) ;
#3827=CARTESIAN_POINT ( 'NONE',  ( -30.00000000000002842, -25.00000000000000000, 200.0000000000000000 ) ) ;
#3847=CARTESIAN_POINT ( 'NONE',  ( -30.00000000000002842, -25.00000000000000000, 200.0000000000000000 ) ) ;
#3857=DIRECTION ( 'NONE',  ( -0.000000000000000000, 1.000000000000000000, -0.000000000000000000 ) ) ;
#3864=CARTESIAN_POINT ( 'NONE',  ( 107.9310344827585908, -20.00000000000000000, -144.8275862068965125 ) ) ;
#3867=ADVANCED_FACE ( 'NONE', ( #5364 ), #7370, .F. ) ;
#3871=LINE ( 'NONE', #3827, #6009 ) ;
#3885=CIRCLE ( 'NONE', #8341, 2.649999999999985700 ) ;
#3891=AXIS2_PLACEMENT_3D ( 'NONE', #6495, #534, #3195 ) ;
#3896=DIRECTION ( 'NONE',  ( 0.000000000000000000, 0.000000000000000000, 1.000000000000000000 ) ) ;
#3898=ORIENTED_EDGE ( 'NONE', *, *, #1735, .T. ) ;
#3904=ADVANCED_FACE ( 'NONE', ( #1450 ), #7233, .F. ) ;
#3905=CARTESIAN_POINT ( 'NONE',  ( 0.000000000000000000, 0.000000000000000000, 200.0000000000000000 ) ) ;
#3911=ORIENTED_EDGE ( 'NONE', *, *, #5222, .F. ) ;
#3921=DIRECTION ( 'NONE',  ( -0.000000000000000000, 1.000000000000000000, -0.000000000000000000 ) ) ;
#3922=ORIENTED_EDGE ( 'NONE', *, *, #5547, .T. ) ;
#3927=FACE_OUTER_BOUND ( 'NONE', #6670, .T. ) ;
#3931=( LENGTH_UNIT ( ) NAMED_UNIT ( * ) SI_UNIT ( .MILLI., .METRE. ) );
#3937=CARTESIAN_POINT ( 'NONE',  ( 470.0000000000000000, -25.00000000000000000, 200.0000000000000000 ) ) ;
#3953=CIRCLE ( 'NONE', #7569, 2.649999999999985700 ) ;
#3958=DIRECTION ( 'NONE',  ( -0.000000000000000000, 1.000000000000000000, -0.000000000000000000 ) ) ;
#3962=ORIENTED_EDGE ( 'NONE', *, *, #3006, .T. ) ;
#3976=VERTEX_POINT ( 'NONE', #6054 ) ;
#3980=CIRCLE ( 'NONE', #2470, 2.649999999999985700 ) ;
#3989=EDGE_CURVE ( 'NONE', #2349, #6369, #2887, .T. ) ;
#3990=ORIENTED_EDGE ( 'NONE', *, *, #8090, .T. ) ;
#3996=PRODUCT_DEFINITION_SHAPE ( 'NONE', 'NONE',  #424 ) ;
#4019=CIRCLE ( 'NONE', #1803, 2.649999999999985700 ) ;
#4026=FACE_OUTER_BOUND ( 'NONE', #7511, .T. ) ;
#4027=EDGE_LOOP ( 'NONE', ( #2212, #6146, #2282, #5992 ) ) ;
#4048=ORIENTED_EDGE ( 'NONE', *, *, #3433, .F. ) ;
#4055=CARTESIAN_POINT ( 'NONE',  ( 386.6666666666666288, -20.00000000000000000, 162.5000000000000853 ) ) ;
#4060=CYLINDRICAL_SURFACE ( 'NONE', #3366, 2.649999999999985700 ) ;
#4069=EDGE_LOOP ( 'NONE', ( #3026, #3962, #1775, #5163 ) ) ;
#4074=CIRCLE ( 'NONE', #8252, 2.649999999999985700 ) ;
#4080=ORIENTED_EDGE ( 'NONE', *, *, #288, .T. ) ;
#4083=CARTESIAN_POINT ( 'NONE',  ( 470.0000000000000000, -19.99999999999979394, 0.000000000000000000 ) ) ;
#4088=ORIENTED_EDGE ( 'NONE', *, *, #1168, .F. ) ;
#4104=ORIENTED_EDGE ( 'NONE', *, *, #2742, .F. ) ;
#4113=CLOSED_SHELL ( 'NONE', ( #742, #1429, #7592, #3867, #4925, #1058, #6100, #6266, #4811, #3904, #8106, #557, #6660, #439, #4440, #1570, #4694, #8286, #7151, #5556, #1169, #397, #3660, #4437, #1864, #2660, #8014, #6028 ) ) ;
#4115=DIRECTION ( 'NONE',  ( -0.000000000000000000, 1.000000000000000000, -0.000000000000000000 ) ) ;
#4122=EDGE_CURVE ( 'NONE', #1609, #4392, #5574, .T. ) ;
#4135=FACE_OUTER_BOUND ( 'NONE', #3360, .T. ) ;
#4137=ORIENTED_EDGE ( 'NONE', *, *, #6722, .F. ) ;
#4142=EDGE_LOOP ( 'NONE', ( #106, #3227, #4486, #7679 ) ) ;
#4148=DIRECTION ( 'NONE',  ( 0.000000000000000000, 0.000000000000000000, 1.000000000000000000 ) ) ;
#4170=CARTESIAN_POINT ( 'NONE',  ( -30.00000000000002842, -25.00000000000000000, -200.0000000000000000 ) ) ;
#4175=CARTESIAN_POINT ( 'NONE',  ( 352.0000000000000000, -20.00000000000000000, -16.23142504031546807 ) ) ;
#4176=ORIENTED_EDGE ( 'NONE', *, *, #6462, .F. ) ;
#4181=LINE ( 'NONE', #4229, #2764 ) ;
#4202=CIRCLE ( 'NONE', #453, 2.649999999999985700 ) ;
#4205=CIRCLE ( 'NONE', #3658, 2.649999999999985700 ) ;
#4229=CARTESIAN_POINT ( 'NONE',  ( 3.245314017740478073E-16, -20.00000000000000000, -160.1500000000000057 ) ) ;
#4240=ORIENTED_EDGE ( 'NONE', *, *, #3038, .F. ) ;
#4251=CARTESIAN_POINT ( 'NONE',  ( 439.9999999999999432, -20.00000000000000000, 18.96857495968446017 ) ) ;
#4264=AXIS2_PLACEMENT_3D ( 'NONE', #417, #6465, #8479 ) ;
#4268=FACE_BOUND ( 'NONE', #4796, .T. ) ;
#4277=CARTESIAN_POINT ( 'NONE',  ( 439.9999999999999432, -20.00000000000000000, 18.96857495968446017 ) ) ;
#4284=EDGE_CURVE ( 'NONE', #6072, #2349, #8208, .T. ) ;
#4293=( LENGTH_UNIT ( ) NAMED_UNIT ( * ) SI_UNIT ( .MILLI., .METRE. ) );
#4302=CARTESIAN_POINT ( 'NONE',  ( 53.33333333333330017, -20.00000000000000000, 162.5000000000000853 ) ) ;
#4305=ORIENTED_EDGE ( 'NONE', *, *, #3989, .T. ) ;
#4319=VERTEX_POINT ( 'NONE', #1060 ) ;
#4320=CYLINDRICAL_SURFACE ( 'NONE', #6143, 2.649999999999985700 ) ;
#4335=CARTESIAN_POINT ( 'NONE',  ( 303.3333333333333144, -20.00000000000000000, 162.5000000000000853 ) ) ;
#4363=ORIENTED_EDGE ( 'NONE', *, *, #7820, .T. ) ;
#4373=ORIENTED_EDGE ( 'NONE', *, *, #8506, .F. ) ;
#4383=DIRECTION ( 'NONE',  ( -0.9284766908852593037, 0.000000000000000000, -0.3713906763541036660 ) ) ;
#4392=VERTEX_POINT ( 'NONE', #8280 ) ;
#4435=ORIENTED_EDGE ( 'NONE', *, *, #5862, .F. ) ;
#4437=ADVANCED_FACE ( 'NONE', ( #8411 ), #7665, .F. ) ;
#4438=CARTESIAN_POINT ( 'NONE',  ( 386.6666666666666288, -20.00000000000000000, 159.8500000000001080 ) ) ;
#4440=ADVANCED_FACE ( 'NONE', ( #1792 ), #5043, .T. ) ;
#4447=AXIS2_PLACEMENT_3D ( 'NONE', #7150, #5795, #1190 ) ;
#4454=ORIENTED_EDGE ( 'NONE', *, *, #5495, .T. ) ;
#4457=CARTESIAN_POINT ( 'NONE',  ( 219.9999999999999716, -20.00000000000000000, 162.5000000000000853 ) ) ;
#4484=ORIENTED_EDGE ( 'NONE', *, *, #7478, .F. ) ;
#4486=ORIENTED_EDGE ( 'NONE', *, *, #1593, .F. ) ;
#4488=CIRCLE ( 'NONE', #6295, 2.649999999999985700 ) ;
#4491=FACE_BOUND ( 'NONE', #3726, .T. ) ;
#4495=EDGE_CURVE ( 'NONE', #8491, #437, #7976, .T. ) ;
#4498=DIRECTION ( 'NONE',  ( -0.000000000000000000, 1.000000000000000000, -0.000000000000000000 ) ) ;
#4508=DIRECTION ( 'NONE',  ( -0.9284766908852593037, 0.000000000000000000, -0.3713906763541036660 ) ) ;
#4513=DIRECTION ( 'NONE',  ( 0.000000000000000000, 0.000000000000000000, 1.000000000000000000 ) ) ;
#4526=AXIS2_PLACEMENT_3D ( 'NONE', #5546, #3768, #5068 ) ;
#4532=AXIS2_PLACEMENT_3D ( 'NONE', #583, #50, #626 ) ;
#4542=ORIENTED_EDGE ( 'NONE', *, *, #745, .F. ) ;
#4572=ORIENTED_EDGE ( 'NONE', *, *, #1844, .T. ) ;
#4582=CARTESIAN_POINT ( 'NONE',  ( 136.6666666666666288, -25.00000000000000000, 162.5000000000000853 ) ) ;
#4588=VECTOR ( 'NONE', #4809, 1000.000000000000000 ) ;
#4593=DIRECTION ( 'NONE',  ( 0.000000000000000000, 0.000000000000000000, 1.000000000000000000 ) ) ;
#4605=EDGE_LOOP ( 'NONE', ( #7321, #7643 ) ) ;
#4620=CARTESIAN_POINT ( 'NONE',  ( -30.00000000000002842, -24.99999999999980105, -200.0000000000000000 ) ) ;
#4624=AXIS2_PLACEMENT_3D ( 'NONE', #1174, #7834, #3345 ) ;
#4663=AXIS2_PLACEMENT_3D ( 'NONE', #4335, #414, #5679 ) ;
#4664=CARTESIAN_POINT ( 'NONE',  ( -30.00000000000002842, -20.00000000000000000, 200.0000000000000000 ) ) ;
#4684=ORIENTED_EDGE ( 'NONE', *, *, #8314, .F. ) ;
#4694=ADVANCED_FACE ( 'NONE', ( #6457 ), #5552, .F. ) ;
#4709=ORIENTED_EDGE ( 'NONE', *, *, #3577, .T. ) ;
#4722=AXIS2_PLACEMENT_3D ( 'NONE', #2719, #8037, #5273 ) ;
#4727=LINE ( 'NONE', #2567, #2463 ) ;
#4736=DIRECTION ( 'NONE',  ( 0.000000000000000000, 0.000000000000000000, 1.000000000000000000 ) ) ;
#4752=DIRECTION ( 'NONE',  ( 0.000000000000000000, 0.000000000000000000, 1.000000000000000000 ) ) ;
#4760=LINE ( 'NONE', #1451, #6373 ) ;
#4769=AXIS2_PLACEMENT_3D ( 'NONE', #7669, #1705, #6441 ) ;
#4793=EDGE_CURVE ( 'NONE', #3710, #8068, #2759, .T. ) ;
#4796=EDGE_LOOP ( 'NONE', ( #7806, #4176 ) ) ;
#4799=CARTESIAN_POINT ( 'NONE',  ( 53.33333333333330017, -20.00000000000000000, 162.5000000000000853 ) ) ;
#4809=DIRECTION ( 'NONE',  ( -0.000000000000000000, 1.000000000000000000, -0.000000000000000000 ) ) ;
#4811=ADVANCED_FACE ( 'NONE', ( #5357 ), #8078, .F. ) ;
#4837=FACE_BOUND ( 'NONE', #382, .T. ) ;
#4841=ORIENTED_EDGE ( 'NONE', *, *, #5439, .T. ) ;
#4844=EDGE_CURVE ( 'NONE', #1160, #702, #6980, .T. ) ;
#4850=CARTESIAN_POINT ( 'NONE',  ( 264.0000000000000000, -20.00000000000000000, -51.43142504031546025 ) ) ;
#4852=VERTEX_POINT ( 'NONE', #4620 ) ;
#4859=LINE ( 'NONE', #2119, #1577 ) ;
#4860=DIRECTION ( 'NONE',  ( 0.000000000000000000, 0.000000000000000000, 1.000000000000000000 ) ) ;
#4864=ORIENTED_EDGE ( 'NONE', *, *, #288, .F. ) ;
#4868=CYLINDRICAL_SURFACE ( 'NONE', #4909, 2.649999999999985700 ) ;
#4869=AXIS2_PLACEMENT_3D ( 'NONE', #2449, #7047, #6392 ) ;
#4873=ORIENTED_EDGE ( 'NONE', *, *, #8369, .F. ) ;
#4909=AXIS2_PLACEMENT_3D ( 'NONE', #151, #1431, #6867 ) ;
#4912=CARTESIAN_POINT ( 'NONE',  ( 3.245314017740487441E-16, -25.00000000000000000, -160.1500000000000057 ) ) ;
#4925=ADVANCED_FACE ( 'NONE', ( #7590 ), #4320, .F. ) ;
#4927=CARTESIAN_POINT ( 'NONE',  ( 303.3333333333333144, -20.00000000000000000, 159.8500000000001080 ) ) ;
#4945=DIRECTION ( 'NONE',  ( 0.000000000000000000, -1.000000000000000000, 0.000000000000000000 ) ) ;
#4947=( LENGTH_UNIT ( ) NAMED_UNIT ( * ) SI_UNIT ( .MILLI., .METRE. ) );
#4957=CARTESIAN_POINT ( 'NONE',  ( 53.33333333333330017, -25.00000000000000000, 162.5000000000000853 ) ) ;
#4959=AXIS2_PLACEMENT_3D ( 'NONE', #6190, #8211, #6365 ) ;
#4965=FACE_BOUND ( 'NONE', #8349, .T. ) ;
#4967=DIRECTION ( 'NONE',  ( -0.000000000000000000, 1.000000000000000000, -0.000000000000000000 ) ) ;
#4972=ORIENTED_EDGE ( 'NONE', *, *, #3989, .F. ) ;
#4992=CARTESIAN_POINT ( 'NONE',  ( 303.3333333333333144, -20.00000000000000000, 159.8500000000001080 ) ) ;
#5001=VERTEX_POINT ( 'NONE', #6842 ) ;
#5003=DIRECTION ( 'NONE',  ( -0.000000000000000000, 1.000000000000000000, -0.000000000000000000 ) ) ;
#5004=CARTESIAN_POINT ( 'NONE',  ( 264.0000000000000000, -20.00000000000000000, -48.78142504031547588 ) ) ;
#5028=( NAMED_UNIT ( * ) PLANE_ANGLE_UNIT ( ) SI_UNIT ( $, .RADIAN. ) );
#5031=VERTEX_POINT ( 'NONE', #3582 ) ;
#5043=PLANE ( 'NONE',  #3756 ) ;
#5049=AXIS2_PLACEMENT_3D ( 'NONE', #7758, #5003, #1795 ) ;
#5057=CARTESIAN_POINT ( 'NONE',  ( 136.6666666666666288, -20.00000000000000000, 159.8500000000001080 ) ) ;
#5068=DIRECTION ( 'NONE',  ( 0.000000000000000000, 0.000000000000000000, 1.000000000000000000 ) ) ;
#5072=CARTESIAN_POINT ( 'NONE',  ( 219.9999999999999716, -20.00000000000000000, 165.1500000000000625 ) ) ;
#5081=CARTESIAN_POINT ( 'NONE',  ( 136.6666666666666288, -20.00000000000000000, 162.5000000000000853 ) ) ;
#5085=EDGE_LOOP ( 'NONE', ( #5802, #3434 ) ) ;
#5114=ORIENTED_EDGE ( 'NONE', *, *, #5888, .T. ) ;
#5130=ORIENTED_EDGE ( 'NONE', *, *, #6116, .T. ) ;
#5133=CARTESIAN_POINT ( 'NONE',  ( -30.00000000000002842, -25.00000000000000000, 200.0000000000000000 ) ) ;
#5137=CYLINDRICAL_SURFACE ( 'NONE', #6230, 2.649999999999985700 ) ;
#5141=VERTEX_POINT ( 'NONE', #1717 ) ;
#5161=EDGE_CURVE ( 'NONE', #8500, #5001, #6698, .T. ) ;
#5163=ORIENTED_EDGE ( 'NONE', *, *, #5888, .F. ) ;
#5188=DIRECTION ( 'NONE',  ( -0.000000000000000000, -0.000000000000000000, -1.000000000000000000 ) ) ;
#5192=DIRECTION ( 'NONE',  ( -0.000000000000000000, 1.000000000000000000, -0.000000000000000000 ) ) ;
#5196=DIRECTION ( 'NONE',  ( 0.000000000000000000, 0.000000000000000000, 1.000000000000000000 ) ) ;
#5216=DIRECTION ( 'NONE',  ( 0.000000000000000000, 0.000000000000000000, 1.000000000000000000 ) ) ;
#5221=DIRECTION ( 'NONE',  ( 0.000000000000000000, 0.000000000000000000, 1.000000000000000000 ) ) ;
#5222=EDGE_CURVE ( 'NONE', #1611, #3710, #8527, .T. ) ;
#5223=AXIS2_PLACEMENT_3D ( 'NONE', #5081, #5808, #8484 ) ;
#5229=CIRCLE ( 'NONE', #4959, 2.649999999999985700 ) ;
#5238=FACE_OUTER_BOUND ( 'NONE', #2580, .T. ) ;
#5241=FACE_OUTER_BOUND ( 'NONE', #6600, .T. ) ;
#5246=CARTESIAN_POINT ( 'NONE',  ( 0.000000000000000000, -20.00000000000000000, -154.8500000000000512 ) ) ;
#5249=ORIENTED_EDGE ( 'NONE', *, *, #5547, .F. ) ;
#5259=VERTEX_POINT ( 'NONE', #6528 ) ;
#5262=EDGE_CURVE ( 'NONE', #7313, #6803, #4074, .T. ) ;
#5263=DIRECTION ( 'NONE',  ( 0.000000000000000000, 0.000000000000000000, 1.000000000000000000 ) ) ;
#5273=DIRECTION ( 'NONE',  ( 0.000000000000000000, 0.000000000000000000, 1.000000000000000000 ) ) ;
#5278=EDGE_LOOP ( 'NONE', ( #1336, #4454 ) ) ;
#5279=EDGE_CURVE ( 'NONE', #5393, #1782, #4488, .T. ) ;
#5287=CARTESIAN_POINT ( 'NONE',  ( 219.9999999999999716, -20.00000000000000000, 159.8500000000001080 ) ) ;
#5306=VECTOR ( 'NONE', #3583, 1000.000000000000000 ) ;
#5315=STYLED_ITEM ( 'NONE', ( #3039 ), #6044 ) ;
#5320=AXIS2_PLACEMENT_3D ( 'NONE', #5716, #3031, #5758 ) ;
#5327=DIRECTION ( 'NONE',  ( 0.000000000000000000, 0.000000000000000000, 1.000000000000000000 ) ) ;
#5351=DIRECTION ( 'NONE',  ( 0.000000000000000000, 1.000000000000000000, 0.000000000000000000 ) ) ;
#5352=AXIS2_PLACEMENT_3D ( 'NONE', #4302, #912, #7480 ) ;
#5357=FACE_OUTER_BOUND ( 'NONE', #2725, .T. ) ;
#5362=CARTESIAN_POINT ( 'NONE',  ( 176.0000000000000000, -20.00000000000000000, -83.98142504031548583 ) ) ;
#5364=FACE_OUTER_BOUND ( 'NONE', #7292, .T. ) ;
#5378=DIRECTION ( 'NONE',  ( 0.000000000000000000, 0.000000000000000000, -1.000000000000000000 ) ) ;
#5388=EDGE_CURVE ( 'NONE', #5393, #590, #8152, .T. ) ;
#5391=ORIENTED_EDGE ( 'NONE', *, *, #2769, .T. ) ;
#5393=VERTEX_POINT ( 'NONE', #6830 ) ;
#5405=VECTOR ( 'NONE', #5188, 1000.000000000000000 ) ;
#5410=ORIENTED_EDGE ( 'NONE', *, *, #235, .T. ) ;
#5428=DIRECTION ( 'NONE',  ( -0.000000000000000000, 1.000000000000000000, -0.000000000000000000 ) ) ;
#5438=CARTESIAN_POINT ( 'NONE',  ( 0.000000000000000000, -20.00000000000000000, -157.5000000000000284 ) ) ;
#5439=EDGE_CURVE ( 'NONE', #7313, #2500, #1833, .T. ) ;
#5441=VERTEX_POINT ( 'NONE', #4438 ) ;
#5467=ORIENTED_EDGE ( 'NONE', *, *, #235, .F. ) ;
#5470=CARTESIAN_POINT ( 'NONE',  ( 219.9999999999999716, -25.00000000000000000, 162.5000000000000853 ) ) ;
#5492=DIRECTION ( 'NONE',  ( 0.000000000000000000, 0.000000000000000000, 1.000000000000000000 ) ) ;
#5495=EDGE_CURVE ( 'NONE', #542, #1660, #6704, .T. ) ;
#5501=EDGE_LOOP ( 'NONE', ( #4709, #7084 ) ) ;
#5511=ORIENTED_EDGE ( 'NONE', *, *, #2023, .T. ) ;
#5523=ORIENTED_EDGE ( 'NONE', *, *, #5995, .T. ) ;
#5546=CARTESIAN_POINT ( 'NONE',  ( 264.0000000000000000, -20.00000000000000000, -51.43142504031546025 ) ) ;
#5547=EDGE_CURVE ( 'NONE', #6181, #437, #387, .T. ) ;
#5552=CYLINDRICAL_SURFACE ( 'NONE', #301, 2.649999999999985700 ) ;
#5556=ADVANCED_FACE ( 'NONE', ( #3179 ), #3054, .F. ) ;
#5558=DIRECTION ( 'NONE',  ( 0.000000000000000000, 0.000000000000000000, 1.000000000000000000 ) ) ;
#5574=LINE ( 'NONE', #2336, #2802 ) ;
#5590=ORIENTED_EDGE ( 'NONE', *, *, #2587, .F. ) ;
#5591=SHAPE_REPRESENTATION_RELATIONSHIP ( 'NONE' , 'NONE' ,  #2707, #6044 ) ;
#5678=VERTEX_POINT ( 'NONE', #1961 ) ;
#5679=DIRECTION ( 'NONE',  ( 0.000000000000000000, 0.000000000000000000, 1.000000000000000000 ) ) ;
#5697=DIRECTION ( 'NONE',  ( -0.000000000000000000, 1.000000000000000000, -0.000000000000000000 ) ) ;
#5707=FACE_BOUND ( 'NONE', #5085, .T. ) ;
#5711=ORIENTED_EDGE ( 'NONE', *, *, #5279, .F. ) ;
#5714=CARTESIAN_POINT ( 'NONE',  ( 386.6666666666666288, -20.00000000000000000, 162.5000000000000853 ) ) ;
#5716=CARTESIAN_POINT ( 'NONE',  ( 176.0000000000000000, -20.00000000000000000, -86.63142504031547730 ) ) ;
#5718=ORIENTED_EDGE ( 'NONE', *, *, #1233, .F. ) ;
#5735=AXIS2_PLACEMENT_3D ( 'NONE', #8005, #5852, #4513 ) ;
#5749=CIRCLE ( 'NONE', #6712, 2.649999999999985700 ) ;
#5751=FACE_BOUND ( 'NONE', #6342, .T. ) ;
#5758=DIRECTION ( 'NONE',  ( 0.000000000000000000, 0.000000000000000000, 1.000000000000000000 ) ) ;
#5762=CARTESIAN_POINT ( 'NONE',  ( 352.0000000000000000, -20.00000000000000000, -16.23142504031546807 ) ) ;
#5764=DIRECTION ( 'NONE',  ( 1.000000000000000000, 0.000000000000000000, 0.000000000000000000 ) ) ;
#5767=ORIENTED_EDGE ( 'NONE', *, *, #2587, .T. ) ;
#5769=EDGE_CURVE ( 'NONE', #5259, #6891, #4205, .T. ) ;
#5776=CARTESIAN_POINT ( 'NONE',  ( -30.00000000000002842, -25.00000000000000000, 200.0000000000000000 ) ) ;
#5782=LINE ( 'NONE', #5004, #8134 ) ;
#5787=CARTESIAN_POINT ( 'NONE',  ( 136.6666666666666288, -20.00000000000000000, 162.5000000000000853 ) ) ;
#5789=EDGE_CURVE ( 'NONE', #6181, #6418, #2825, .T. ) ;
#5795=DIRECTION ( 'NONE',  ( 0.000000000000000000, 1.000000000000000000, 0.000000000000000000 ) ) ;
#5798=EDGE_CURVE ( 'NONE', #7972, #7459, #1469, .T. ) ;
#5802=ORIENTED_EDGE ( 'NONE', *, *, #5789, .T. ) ;
#5805=PLANE ( 'NONE',  #6318 ) ;
#5808=DIRECTION ( 'NONE',  ( -0.000000000000000000, 1.000000000000000000, -0.000000000000000000 ) ) ;
#5831=CARTESIAN_POINT ( 'NONE',  ( 470.0000000000000000, -20.00000000000000000, 200.0000000000000000 ) ) ;
#5838=DIRECTION ( 'NONE',  ( -0.000000000000000000, 1.000000000000000000, -0.000000000000000000 ) ) ;
#5852=DIRECTION ( 'NONE',  ( 0.000000000000000000, 1.000000000000000000, 0.000000000000000000 ) ) ;
#5862=EDGE_CURVE ( 'NONE', #6418, #8491, #7079, .T. ) ;
#5878=( NAMED_UNIT ( * ) PLANE_ANGLE_UNIT ( ) SI_UNIT ( $, .RADIAN. ) );
#5880=DIRECTION ( 'NONE',  ( -0.000000000000000000, 1.000000000000000000, -0.000000000000000000 ) ) ;
#5882=CARTESIAN_POINT ( 'NONE',  ( 386.6666666666666288, -25.00000000000000000, 162.5000000000000853 ) ) ;
#5883=VECTOR ( 'NONE', #1663, 1000.000000000000000 ) ;
#5885=CARTESIAN_POINT ( 'NONE',  ( 88.00000000000000000, -20.00000000000000000, -121.8314250403154659 ) ) ;
#5888=EDGE_CURVE ( 'NONE', #6119, #8049, #7784, .T. ) ;
#5905=DIRECTION ( 'NONE',  ( -0.000000000000000000, 1.000000000000000000, -0.000000000000000000 ) ) ;
#5906=DIRECTION ( 'NONE',  ( -0.000000000000000000, 1.000000000000000000, -0.000000000000000000 ) ) ;
#5912=DIRECTION ( 'NONE',  ( -0.000000000000000000, 1.000000000000000000, -0.000000000000000000 ) ) ;
#5916=CARTESIAN_POINT ( 'NONE',  ( 53.33333333333330017, -25.00000000000000000, 159.8500000000001080 ) ) ;
#5926=DIRECTION ( 'NONE',  ( -0.000000000000000000, 1.000000000000000000, -0.000000000000000000 ) ) ;
#5928=VERTEX_POINT ( 'NONE', #3044 ) ;
#5930=( GEOMETRIC_REPRESENTATION_CONTEXT ( 3 ) GLOBAL_UNCERTAINTY_ASSIGNED_CONTEXT ( ( #7938 ) ) GLOBAL_UNIT_ASSIGNED_CONTEXT ( ( #3931, #5878, #7937 ) ) REPRESENTATION_CONTEXT ( 'NONE', 'WORKASPACE' ) );
#5932=DIRECTION ( 'NONE',  ( -0.9284766908852593037, 0.000000000000000000, -0.3713906763541036660 ) ) ;
#5944=AXIS2_PLACEMENT_3D ( 'NONE', #8584, #1965, #7971 ) ;
#5948=VECTOR ( 'NONE', #3857, 1000.000000000000000 ) ;
#5949=DIRECTION ( 'NONE',  ( 0.000000000000000000, 0.000000000000000000, 1.000000000000000000 ) ) ;
#5977=CARTESIAN_POINT ( 'NONE',  ( 88.00000000000000000, -20.00000000000000000, -121.8314250403154659 ) ) ;
#5992=ORIENTED_EDGE ( 'NONE', *, *, #1593, .T. ) ;
#5995=EDGE_CURVE ( 'NONE', #1878, #7699, #8000, .T. ) ;
#5997=CARTESIAN_POINT ( 'NONE',  ( 53.33333333333330017, -25.00000000000000000, 162.5000000000000853 ) ) ;
#6001=DIRECTION ( 'NONE',  ( 0.000000000000000000, 0.000000000000000000, 1.000000000000000000 ) ) ;
#6002=CARTESIAN_POINT ( 'NONE',  ( 470.0000000000000000, 786.6649314574284517, 0.000000000000000000 ) ) ;
#6006=CARTESIAN_POINT ( 'NONE',  ( 53.33333333333330017, -20.00000000000000000, 159.8500000000001080 ) ) ;
#6008=CIRCLE ( 'NONE', #6438, 2.649999999999985700 ) ;
#6009=VECTOR ( 'NONE', #6473, 1000.000000000000000 ) ;
#6028=ADVANCED_FACE ( 'NONE', ( #6468 ), #5805, .T. ) ;
#6043=EDGE_CURVE ( 'NONE', #101, #5678, #1207, .T. ) ;
#6044=ADVANCED_BREP_SHAPE_REPRESENTATION ( '', ( #2263, #594 ), #6566 ) ;
#6054=CARTESIAN_POINT ( 'NONE',  ( 439.9999999999999432, -20.00000000000000000, 21.61857495968444454 ) ) ;
#6065=ORIENTED_EDGE ( 'NONE', *, *, #1931, .F. ) ;
#6072=VERTEX_POINT ( 'NONE', #6590 ) ;
#6073=DIRECTION ( 'NONE',  ( 0.000000000000000000, 1.000000000000000000, 0.000000000000000000 ) ) ;
#6085=DIRECTION ( 'NONE',  ( -0.000000000000000000, 1.000000000000000000, -0.000000000000000000 ) ) ;
#6098=ORIENTED_EDGE ( 'NONE', *, *, #7478, .T. ) ;
#6100=ADVANCED_FACE ( 'NONE', ( #5241 ), #1947, .F. ) ;
#6102=FACE_OUTER_BOUND ( 'NONE', #4069, .T. ) ;
#6106=LINE ( 'NONE', #6859, #1616 ) ;
#6109=AXIS2_PLACEMENT_3D ( 'NONE', #635, #3291, #2640 ) ;
#6116=EDGE_CURVE ( 'NONE', #6803, #5031, #8044, .T. ) ;
#6117=LINE ( 'NONE', #4170, #3005 ) ;
#6119=VERTEX_POINT ( 'NONE', #6804 ) ;
#6133=EDGE_LOOP ( 'NONE', ( #7737, #2516, #7917, #5249 ) ) ;
#6143=AXIS2_PLACEMENT_3D ( 'NONE', #219, #2973, #2236 ) ;
#6146=ORIENTED_EDGE ( 'NONE', *, *, #6880, .F. ) ;
#6149=EDGE_LOOP ( 'NONE', ( #4972, #8281, #228, #4080 ) ) ;
#6175=ORIENTED_EDGE ( 'NONE', *, *, #7731, .T. ) ;
#6181=VERTEX_POINT ( 'NONE', #6718 ) ;
#6190=CARTESIAN_POINT ( 'NONE',  ( 176.0000000000000000, -25.00000000000000000, -86.63142504031547730 ) ) ;
#6193=AXIS2_PLACEMENT_3D ( 'NONE', #6637, #6594, #4593 ) ;
#6197=CARTESIAN_POINT ( 'NONE',  ( 176.0000000000000000, -20.00000000000000000, -86.63142504031547730 ) ) ;
#6230=AXIS2_PLACEMENT_3D ( 'NONE', #5787, #3707, #8460 ) ;
#6233=EDGE_CURVE ( 'NONE', #6369, #3976, #5749, .T. ) ;
#6252=ORIENTED_EDGE ( 'NONE', *, *, #5388, .T. ) ;
#6264=LINE ( 'NONE', #2964, #5883 ) ;
#6266=ADVANCED_FACE ( 'NONE', ( #6102 ), #3549, .F. ) ;
#6284=CIRCLE ( 'NONE', #587, 2.649999999999985700 ) ;
#6286=DIRECTION ( 'NONE',  ( 0.000000000000000000, 1.000000000000000000, 0.000000000000000000 ) ) ;
#6295=AXIS2_PLACEMENT_3D ( 'NONE', #7931, #7269, #79 ) ;
#6302=ORIENTED_EDGE ( 'NONE', *, *, #4793, .T. ) ;
#6305=DIRECTION ( 'NONE',  ( -1.000000000000000000, 0.000000000000000000, 0.000000000000000000 ) ) ;
#6318=AXIS2_PLACEMENT_3D ( 'NONE', #6508, #3210, #4508 ) ;
#6327=CARTESIAN_POINT ( 'NONE',  ( 219.9999999999999716, -25.00000000000000000, 159.8500000000001080 ) ) ;
#6331=DIRECTION ( 'NONE',  ( -0.000000000000000000, 1.000000000000000000, -0.000000000000000000 ) ) ;
#6332=ORIENTED_EDGE ( 'NONE', *, *, #6719, .F. ) ;
#6342=EDGE_LOOP ( 'NONE', ( #7935, #7014 ) ) ;
#6350=CARTESIAN_POINT ( 'NONE',  ( 386.6666666666666288, -25.00000000000000000, 159.8500000000001080 ) ) ;
#6356=ORIENTED_EDGE ( 'NONE', *, *, #5161, .F. ) ;
#6365=DIRECTION ( 'NONE',  ( 0.000000000000000000, 0.000000000000000000, 1.000000000000000000 ) ) ;
#6369=VERTEX_POINT ( 'NONE', #6413 ) ;
#6373=VECTOR ( 'NONE', #5926, 1000.000000000000000 ) ;
#6379=( NAMED_UNIT ( * ) SI_UNIT ( $, .STERADIAN. ) SOLID_ANGLE_UNIT ( ) );
#6392=DIRECTION ( 'NONE',  ( 0.000000000000000000, 0.000000000000000000, 1.000000000000000000 ) ) ;
#6394=ORIENTED_EDGE ( 'NONE', *, *, #1168, .T. ) ;
#6400=ORIENTED_EDGE ( 'NONE', *, *, #1762, .T. ) ;
#6404=DIRECTION ( 'NONE',  ( 0.000000000000000000, 1.000000000000000000, 0.000000000000000000 ) ) ;
#6411=CARTESIAN_POINT ( 'NONE',  ( 439.9999999999999432, -20.00000000000000000, 18.96857495968446017 ) ) ;
#6413=CARTESIAN_POINT ( 'NONE',  ( 439.9999999999999432, -20.00000000000000000, 16.31857495968447225 ) ) ;
#6418=VERTEX_POINT ( 'NONE', #6327 ) ;
#6438=AXIS2_PLACEMENT_3D ( 'NONE', #7081, #2484, #6469 ) ;
#6439=EDGE_LOOP ( 'NONE', ( #4484, #6065 ) ) ;
#6440=MECHANICAL_DESIGN_GEOMETRIC_PRESENTATION_REPRESENTATION('',(#5315),#7551);
#6441=DIRECTION ( 'NONE',  ( 0.000000000000000000, 0.000000000000000000, 1.000000000000000000 ) ) ;
#6457=FACE_OUTER_BOUND ( 'NONE', #6149, .T. ) ;
#6462=EDGE_CURVE ( 'NONE', #7349, #590, #3953, .T. ) ;
#6465=DIRECTION ( 'NONE',  ( -0.000000000000000000, 1.000000000000000000, -0.000000000000000000 ) ) ;
#6467=ORIENTED_EDGE ( 'NONE', *, *, #8369, .T. ) ;
#6468=FACE_OUTER_BOUND ( 'NONE', #7586, .T. ) ;
#6469=DIRECTION ( 'NONE',  ( 0.000000000000000000, 0.000000000000000000, 1.000000000000000000 ) ) ;
#6473=DIRECTION ( 'NONE',  ( 1.000000000000000000, 0.000000000000000000, 0.000000000000000000 ) ) ;
#6479=CIRCLE ( 'NONE', #6193, 2.649999999999985700 ) ;
#6480=DIRECTION ( 'NONE',  ( -0.000000000000000000, 1.000000000000000000, -0.000000000000000000 ) ) ;
#6483=CARTESIAN_POINT ( 'NONE',  ( 470.0000000000000000, -24.99999999999980105, 0.000000000000000000 ) ) ;
#6486=AXIS2_PLACEMENT_3D ( 'NONE', #7742, #8516, #3207 ) ;
#6495=CARTESIAN_POINT ( 'NONE',  ( 176.0000000000000000, -25.00000000000000000, -86.63142504031547730 ) ) ;
#6505=FACE_OUTER_BOUND ( 'NONE', #8433, .T. ) ;
#6508=CARTESIAN_POINT ( 'NONE',  ( -30.00000000000002842, 786.6649314574284517, -200.0000000000000000 ) ) ;
#6518=VERTEX_POINT ( 'NONE', #3937 ) ;
#6528=CARTESIAN_POINT ( 'NONE',  ( 386.6666666666666288, -25.00000000000000000, 165.1500000000000625 ) ) ;
#6538=DIRECTION ( 'NONE',  ( 0.000000000000000000, 1.000000000000000000, 0.000000000000000000 ) ) ;
#6566=( GEOMETRIC_REPRESENTATION_CONTEXT ( 3 ) GLOBAL_UNCERTAINTY_ASSIGNED_CONTEXT ( ( #7997 ) ) GLOBAL_UNIT_ASSIGNED_CONTEXT ( ( #4947, #2942, #6986 ) ) REPRESENTATION_CONTEXT ( 'NONE', 'WORKASPACE' ) );
#6572=CARTESIAN_POINT ( 'NONE',  ( 53.33333333333330017, -20.00000000000000000, 162.5000000000000853 ) ) ;
#6590=CARTESIAN_POINT ( 'NONE',  ( 439.9999999999999432, -25.00000000000000000, 21.61857495968444454 ) ) ;
#6594=DIRECTION ( 'NONE',  ( 0.000000000000000000, 1.000000000000000000, 0.000000000000000000 ) ) ;
#6596=DIRECTION ( 'NONE',  ( 0.000000000000000000, 0.000000000000000000, 1.000000000000000000 ) ) ;
#6600=EDGE_LOOP ( 'NONE', ( #7697, #4841, #8354, #2384 ) ) ;
#6603=CARTESIAN_POINT ( 'NONE',  ( 352.0000000000000000, -20.00000000000000000, -13.58142504031548192 ) ) ;
#6608=ORIENTED_EDGE ( 'NONE', *, *, #6043, .F. ) ;
#6612=CIRCLE ( 'NONE', #929, 2.649999999999985700 ) ;
#6622=DIRECTION ( 'NONE',  ( 0.000000000000000000, 1.000000000000000000, 0.000000000000000000 ) ) ;
#6632=ORIENTED_EDGE ( 'NONE', *, *, #1839, .F. ) ;
#6637=CARTESIAN_POINT ( 'NONE',  ( 264.0000000000000000, -25.00000000000000000, -51.43142504031546025 ) ) ;
#6654=CARTESIAN_POINT ( 'NONE',  ( 0.000000000000000000, -20.00000000000000000, -157.5000000000000284 ) ) ;
#6660=ADVANCED_FACE ( 'NONE', ( #2836, #8285, #2276, #4268, #921, #8196, #8153, #4965, #4837, #2021, #878, #2323 ), #7489, .T. ) ;
#6670=EDGE_LOOP ( 'NONE', ( #790, #6302, #6394, #645 ) ) ;
#6676=FACE_OUTER_BOUND ( 'NONE', #3503, .T. ) ;
#6698=CIRCLE ( 'NONE', #871, 2.649999999999985700 ) ;
#6704=CIRCLE ( 'NONE', #4769, 2.649999999999985700 ) ;
#6706=CIRCLE ( 'NONE', #2966, 2.649999999999985700 ) ;
#6709=AXIS2_PLACEMENT_3D ( 'NONE', #3630, #6286, #3723 ) ;
#6712=AXIS2_PLACEMENT_3D ( 'NONE', #1458, #4115, #2076 ) ;
#6718=CARTESIAN_POINT ( 'NONE',  ( 219.9999999999999716, -25.00000000000000000, 165.1500000000000625 ) ) ;
#6719=EDGE_CURVE ( 'NONE', #4392, #4319, #6918, .T. ) ;
#6722=EDGE_CURVE ( 'NONE', #6999, #1077, #6264, .T. ) ;
#6740=CARTESIAN_POINT ( 'NONE',  ( 386.6666666666666288, -20.00000000000000000, 159.8500000000001080 ) ) ;
#6741=ORIENTED_EDGE ( 'NONE', *, *, #5798, .T. ) ;
#6742=ORIENTED_EDGE ( 'NONE', *, *, #2829, .F. ) ;
#6753=CIRCLE ( 'NONE', #1339, 2.649999999999985700 ) ;
#6756=AXIS2_PLACEMENT_3D ( 'NONE', #5885, #5838, #1982 ) ;
#6759=AXIS2_PLACEMENT_3D ( 'NONE', #3847, #6404, #2506 ) ;
#6767=ORIENTED_EDGE ( 'NONE', *, *, #1684, .F. ) ;
#6770=DIRECTION ( 'NONE',  ( -0.000000000000000000, 1.000000000000000000, -0.000000000000000000 ) ) ;
#6774=ORIENTED_EDGE ( 'NONE', *, *, #5995, .F. ) ;
#6779=CYLINDRICAL_SURFACE ( 'NONE', #7165, 2.649999999999985700 ) ;
#6784=DIRECTION ( 'NONE',  ( -0.000000000000000000, 1.000000000000000000, -0.000000000000000000 ) ) ;
#6789=CARTESIAN_POINT ( 'NONE',  ( 136.6666666666666288, -20.00000000000000000, 162.5000000000000853 ) ) ;
#6803=VERTEX_POINT ( 'NONE', #1219 ) ;
#6804=CARTESIAN_POINT ( 'NONE',  ( 176.0000000000000000, -25.00000000000000000, -83.98142504031548583 ) ) ;
#6809=VERTEX_POINT ( 'NONE', #6483 ) ;
#6830=CARTESIAN_POINT ( 'NONE',  ( 303.3333333333333144, -25.00000000000000000, 165.1500000000000625 ) ) ;
#6842=CARTESIAN_POINT ( 'NONE',  ( 3.245314017740480046E-16, -20.00000000000000000, -160.1500000000000057 ) ) ;
#6843=AXIS2_PLACEMENT_3D ( 'NONE', #3364, #2102, #4752 ) ;
#6859=CARTESIAN_POINT ( 'NONE',  ( -30.00000000000002842, -20.00000000000000000, 200.0000000000000000 ) ) ;
#6867=DIRECTION ( 'NONE',  ( 0.000000000000000000, 0.000000000000000000, 1.000000000000000000 ) ) ;
#6868=AXIS2_PLACEMENT_3D ( 'NONE', #4664, #7326, #1528 ) ;
#6880=EDGE_CURVE ( 'NONE', #1609, #4852, #1134, .T. ) ;
#6884=EDGE_CURVE ( 'NONE', #1660, #678, #5782, .T. ) ;
#6891=VERTEX_POINT ( 'NONE', #6350 ) ;
#6894=ORIENTED_EDGE ( 'NONE', *, *, #2810, .F. ) ;
#6901=DIRECTION ( 'NONE',  ( -0.000000000000000000, 1.000000000000000000, -0.000000000000000000 ) ) ;
#6917=STYLED_ITEM('',(#8643),#2263);
#6918=LINE ( 'NONE', #965, #3539 ) ;
#6950=CARTESIAN_POINT ( 'NONE',  ( 88.00000000000000000, -25.00000000000000000, -124.4814250403154574 ) ) ;
#6958=ORIENTED_EDGE ( 'NONE', *, *, #6884, .F. ) ;
#6970=CARTESIAN_POINT ( 'NONE',  ( 439.9999999999999432, -20.00000000000000000, 16.31857495968447225 ) ) ;
#6980=CIRCLE ( 'NONE', #1285, 2.649999999999985700 ) ;
#6986=( NAMED_UNIT ( * ) SI_UNIT ( $, .STERADIAN. ) SOLID_ANGLE_UNIT ( ) );
#6990=VECTOR ( 'NONE', #6480, 1000.000000000000000 ) ;
#6999=VERTEX_POINT ( 'NONE', #1388 ) ;
#7014=ORIENTED_EDGE ( 'NONE', *, *, #4844, .T. ) ;
#7016=DIRECTION ( 'NONE',  ( -0.000000000000000000, 1.000000000000000000, -0.000000000000000000 ) ) ;
#7047=DIRECTION ( 'NONE',  ( -0.000000000000000000, 1.000000000000000000, -0.000000000000000000 ) ) ;
#7079=LINE ( 'NONE', #1124, #171 ) ;
#7081=CARTESIAN_POINT ( 'NONE',  ( 303.3333333333333144, -25.00000000000000000, 162.5000000000000853 ) ) ;
#7084=ORIENTED_EDGE ( 'NONE', *, *, #2112, .T. ) ;
#7088=ORIENTED_EDGE ( 'NONE', *, *, #6884, .T. ) ;
#7110=PRODUCT_DEFINITION_FORMATION_WITH_SPECIFIED_SOURCE ( 'ANY', '', #8034, .NOT_KNOWN. ) ;
#7113=ORIENTED_EDGE ( 'NONE', *, *, #3133, .T. ) ;
#7116=VECTOR ( 'NONE', #843, 1000.000000000000000 ) ;
#7119=ORIENTED_EDGE ( 'NONE', *, *, #30, .F. ) ;
#7128=ORIENTED_EDGE ( 'NONE', *, *, #8436, .T. ) ;
#7135=CIRCLE ( 'NONE', #5735, 2.649999999999985700 ) ;
#7149=FACE_BOUND ( 'NONE', #5278, .T. ) ;
#7150=CARTESIAN_POINT ( 'NONE',  ( 439.9999999999999432, -25.00000000000000000, 18.96857495968446017 ) ) ;
#7151=ADVANCED_FACE ( 'NONE', ( #2950 ), #4868, .F. ) ;
#7161=CYLINDRICAL_SURFACE ( 'NONE', #4264, 2.649999999999985700 ) ;
#7165=AXIS2_PLACEMENT_3D ( 'NONE', #995, #5428, #5558 ) ;
#7172=ORIENTED_EDGE ( 'NONE', *, *, #30, .T. ) ;
#7187=DIRECTION ( 'NONE',  ( -0.000000000000000000, 1.000000000000000000, -0.000000000000000000 ) ) ;
#7207=ORIENTED_EDGE ( 'NONE', *, *, #4793, .F. ) ;
#7233=CYLINDRICAL_SURFACE ( 'NONE', #7788, 2.649999999999985700 ) ;
#7241=CARTESIAN_POINT ( 'NONE',  ( 136.6666666666666288, -20.00000000000000000, 162.5000000000000853 ) ) ;
#7242=DIRECTION ( 'NONE',  ( 0.000000000000000000, 0.000000000000000000, 1.000000000000000000 ) ) ;
#7263=DIRECTION ( 'NONE',  ( 0.000000000000000000, 0.000000000000000000, 1.000000000000000000 ) ) ;
#7265=VECTOR ( 'NONE', #6784, 1000.000000000000000 ) ;
#7269=DIRECTION ( 'NONE',  ( 0.000000000000000000, 1.000000000000000000, 0.000000000000000000 ) ) ;
#7292=EDGE_LOOP ( 'NONE', ( #969, #8461, #292, #1283 ) ) ;
#7311=VECTOR ( 'NONE', #4945, 1000.000000000000000 ) ;
#7313=VERTEX_POINT ( 'NONE', #6950 ) ;
#7321=ORIENTED_EDGE ( 'NONE', *, *, #2742, .T. ) ;
#7326=DIRECTION ( 'NONE',  ( 0.000000000000000000, 1.000000000000000000, 0.000000000000000000 ) ) ;
#7349=VERTEX_POINT ( 'NONE', #4992 ) ;
#7360=EDGE_CURVE ( 'NONE', #1782, #5393, #6008, .T. ) ;
#7361=DIRECTION ( 'NONE',  ( -0.000000000000000000, 1.000000000000000000, -0.000000000000000000 ) ) ;
#7368=LINE ( 'NONE', #2760, #7116 ) ;
#7370=CYLINDRICAL_SURFACE ( 'NONE', #4722, 2.649999999999985700 ) ;
#7380=ORIENTED_EDGE ( 'NONE', *, *, #745, .T. ) ;
#7382=ORIENTED_EDGE ( 'NONE', *, *, #6233, .F. ) ;
#7426=CARTESIAN_POINT ( 'NONE',  ( -30.00000000000002842, -25.00000000000000000, 200.0000000000000000 ) ) ;
#7446=DIRECTION ( 'NONE',  ( 0.000000000000000000, 0.000000000000000000, 1.000000000000000000 ) ) ;
#7453=DIRECTION ( 'NONE',  ( -0.000000000000000000, 1.000000000000000000, -0.000000000000000000 ) ) ;
#7459=VERTEX_POINT ( 'NONE', #1909 ) ;
#7468=ORIENTED_EDGE ( 'NONE', *, *, #6233, .T. ) ;
#7477=DIRECTION ( 'NONE',  ( -0.000000000000000000, 1.000000000000000000, -0.000000000000000000 ) ) ;
#7478=EDGE_CURVE ( 'NONE', #5031, #2500, #6706, .T. ) ;
#7480=DIRECTION ( 'NONE',  ( 0.000000000000000000, 0.000000000000000000, 1.000000000000000000 ) ) ;
#7484=CIRCLE ( 'NONE', #7634, 2.649999999999985700 ) ;
#7488=CARTESIAN_POINT ( 'NONE',  ( 303.3333333333333144, -20.00000000000000000, 165.1500000000000625 ) ) ;
#7489=PLANE ( 'NONE',  #6868 ) ;
#7507=ORIENTED_EDGE ( 'NONE', *, *, #8090, .F. ) ;
#7511=EDGE_LOOP ( 'NONE', ( #4435, #1729, #3922, #2529 ) ) ;
#7521=DIRECTION ( 'NONE',  ( 0.000000000000000000, 0.000000000000000000, 1.000000000000000000 ) ) ;
#7548=DIRECTION ( 'NONE',  ( -0.000000000000000000, 1.000000000000000000, -0.000000000000000000 ) ) ;
#7551=( GEOMETRIC_REPRESENTATION_CONTEXT ( 3 ) GLOBAL_UNCERTAINTY_ASSIGNED_CONTEXT ( ( #1369 ) ) GLOBAL_UNIT_ASSIGNED_CONTEXT ( ( #4293, #5028, #6379 ) ) REPRESENTATION_CONTEXT ( 'NONE', 'WORKASPACE' ) );
#7559=AXIS2_PLACEMENT_3D ( 'NONE', #4457, #2343, #1112 ) ;
#7562=CARTESIAN_POINT ( 'NONE',  ( 264.0000000000000000, -25.00000000000000000, -48.78142504031547588 ) ) ;
#7569=AXIS2_PLACEMENT_3D ( 'NONE', #8553, #5192, #3812 ) ;
#7575=DIRECTION ( 'NONE',  ( -0.000000000000000000, 1.000000000000000000, -0.000000000000000000 ) ) ;
#7579=VERTEX_POINT ( 'NONE', #2111 ) ;
#7586=EDGE_LOOP ( 'NONE', ( #8270, #5410, #558, #6608 ) ) ;
#7590=FACE_OUTER_BOUND ( 'NONE', #74, .T. ) ;
#7592=ADVANCED_FACE ( 'NONE', ( #770 ), #7648, .F. ) ;
#7603=CARTESIAN_POINT ( 'NONE',  ( 136.6666666666666288, -20.00000000000000000, 165.1500000000000625 ) ) ;
#7607=ORIENTED_EDGE ( 'NONE', *, *, #1844, .F. ) ;
#7625=VECTOR ( 'NONE', #7361, 1000.000000000000000 ) ;
#7634=AXIS2_PLACEMENT_3D ( 'NONE', #3310, #3921, #5949 ) ;
#7643=ORIENTED_EDGE ( 'NONE', *, *, #5262, .T. ) ;
#7648=CYLINDRICAL_SURFACE ( 'NONE', #7559, 2.649999999999985700 ) ;
#7650=CIRCLE ( 'NONE', #3891, 2.649999999999985700 ) ;
#7658=EDGE_CURVE ( 'NONE', #997, #8049, #469, .T. ) ;
#7665=CYLINDRICAL_SURFACE ( 'NONE', #4869, 2.649999999999985700 ) ;
#7667=ORIENTED_EDGE ( 'NONE', *, *, #4122, .F. ) ;
#7669=CARTESIAN_POINT ( 'NONE',  ( 264.0000000000000000, -25.00000000000000000, -51.43142504031546025 ) ) ;
#7679=ORIENTED_EDGE ( 'NONE', *, *, #6719, .T. ) ;
#7697=ORIENTED_EDGE ( 'NONE', *, *, #5262, .F. ) ;
#7699=VERTEX_POINT ( 'NONE', #7603 ) ;
#7716=DIRECTION ( 'NONE',  ( -0.000000000000000000, 1.000000000000000000, -0.000000000000000000 ) ) ;
#7721=FACE_OUTER_BOUND ( 'NONE', #295, .T. ) ;
#7731=EDGE_CURVE ( 'NONE', #6999, #7972, #1869, .T. ) ;
#7733=DIRECTION ( 'NONE',  ( -0.000000000000000000, 1.000000000000000000, -0.000000000000000000 ) ) ;
#7737=ORIENTED_EDGE ( 'NONE', *, *, #7897, .F. ) ;
#7742=CARTESIAN_POINT ( 'NONE',  ( 470.0000000000000000, -20.00000000000000000, 200.0000000000000000 ) ) ;
#7744=EDGE_LOOP ( 'NONE', ( #5467, #3004, #8137, #2242 ) ) ;
#7758=CARTESIAN_POINT ( 'NONE',  ( 176.0000000000000000, -20.00000000000000000, -86.63142504031547730 ) ) ;
#7778=CARTESIAN_POINT ( 'NONE',  ( 303.3333333333333144, -25.00000000000000000, 159.8500000000001080 ) ) ;
#7784=LINE ( 'NONE', #2310, #499 ) ;
#7788=AXIS2_PLACEMENT_3D ( 'NONE', #1404, #3367, #2 ) ;
#7806=ORIENTED_EDGE ( 'NONE', *, *, #1762, .F. ) ;
#7820=EDGE_CURVE ( 'NONE', #6891, #5259, #4202, .T. ) ;
#7824=ORIENTED_EDGE ( 'NONE', *, *, #3036, .T. ) ;
#7834=DIRECTION ( 'NONE',  ( -0.000000000000000000, 1.000000000000000000, -0.000000000000000000 ) ) ;
#7867=VECTOR ( 'NONE', #825, 1000.000000000000000 ) ;
#7868=DIRECTION ( 'NONE',  ( -0.000000000000000000, 1.000000000000000000, -0.000000000000000000 ) ) ;
#7882=CARTESIAN_POINT ( 'NONE',  ( 88.00000000000000000, -25.00000000000000000, -121.8314250403154659 ) ) ;
#7897=EDGE_CURVE ( 'NONE', #6418, #6181, #6284, .T. ) ;
#7906=ORIENTED_EDGE ( 'NONE', *, *, #794, .F. ) ;
#7917=ORIENTED_EDGE ( 'NONE', *, *, #4495, .T. ) ;
#7921=APPLICATION_CONTEXT ( 'automotive_design' ) ;
#7931=CARTESIAN_POINT ( 'NONE',  ( 303.3333333333333144, -25.00000000000000000, 162.5000000000000853 ) ) ;
#7935=ORIENTED_EDGE ( 'NONE', *, *, #1839, .T. ) ;
#7937=( NAMED_UNIT ( * ) SI_UNIT ( $, .STERADIAN. ) SOLID_ANGLE_UNIT ( ) );
#7938=UNCERTAINTY_MEASURE_WITH_UNIT (LENGTH_MEASURE( 1.000000000000000082E-05 ), #3931, 'distance_accuracy_value', 'NONE');
#7939=CARTESIAN_POINT ( 'NONE',  ( 0.000000000000000000, -25.00000000000000000, -157.5000000000000284 ) ) ;
#7951=DIRECTION ( 'NONE',  ( -0.000000000000000000, 1.000000000000000000, -0.000000000000000000 ) ) ;
#7968=AXIS2_PLACEMENT_3D ( 'NONE', #4277, #7016, #1718 ) ;
#7971=DIRECTION ( 'NONE',  ( 0.000000000000000000, 0.000000000000000000, 1.000000000000000000 ) ) ;
#7972=VERTEX_POINT ( 'NONE', #45 ) ;
#7976=CIRCLE ( 'NONE', #4624, 2.649999999999985700 ) ;
#7979=EDGE_CURVE ( 'NONE', #6518, #6809, #7368, .T. ) ;
#7982=CARTESIAN_POINT ( 'NONE',  ( 439.9999999999999432, -20.00000000000000000, 21.61857495968444454 ) ) ;
#7997=UNCERTAINTY_MEASURE_WITH_UNIT (LENGTH_MEASURE( 1.000000000000000082E-05 ), #4947, 'distance_accuracy_value', 'NONE');
#8000=CIRCLE ( 'NONE', #196, 2.649999999999985700 ) ;
#8005=CARTESIAN_POINT ( 'NONE',  ( 136.6666666666666288, -25.00000000000000000, 162.5000000000000853 ) ) ;
#8006=CARTESIAN_POINT ( 'NONE',  ( 386.6666666666666288, -20.00000000000000000, 165.1500000000000625 ) ) ;
#8014=ADVANCED_FACE ( 'NONE', ( #2151 ), #4060, .F. ) ;
#8024=DIRECTION ( 'NONE',  ( 0.000000000000000000, 0.000000000000000000, 1.000000000000000000 ) ) ;
#8026=CIRCLE ( 'NONE', #511, 2.649999999999985700 ) ;
#8034=PRODUCT ( 'base plate', 'base plate', '', ( #1512 ) ) ;
#8037=DIRECTION ( 'NONE',  ( -0.000000000000000000, 1.000000000000000000, -0.000000000000000000 ) ) ;
#8044=LINE ( 'NONE', #769, #4588 ) ;
#8049=VERTEX_POINT ( 'NONE', #5362 ) ;
#8068=VERTEX_POINT ( 'NONE', #1540 ) ;
#8078=CYLINDRICAL_SURFACE ( 'NONE', #6843, 2.649999999999985700 ) ;
#8090=EDGE_CURVE ( 'NONE', #5141, #1878, #8249, .T. ) ;
#8106=ADVANCED_FACE ( 'NONE', ( #8379 ), #3622, .F. ) ;
#8134=VECTOR ( 'NONE', #5697, 1000.000000000000000 ) ;
#8137=ORIENTED_EDGE ( 'NONE', *, *, #8436, .F. ) ;
#8144=CARTESIAN_POINT ( 'NONE',  ( 352.0000000000000000, -20.00000000000000000, -18.88142504031545243 ) ) ;
#8152=LINE ( 'NONE', #7488, #1019 ) ;
#8153=FACE_BOUND ( 'NONE', #6439, .T. ) ;
#8156=CARTESIAN_POINT ( 'NONE',  ( 88.00000000000000000, -20.00000000000000000, -124.4814250403154574 ) ) ;
#8160=CIRCLE ( 'NONE', #6756, 2.649999999999985700 ) ;
#8161=VECTOR ( 'NONE', #4383, 1000.000000000000114 ) ;
#8177=ORIENTED_EDGE ( 'NONE', *, *, #2829, .T. ) ;
#8196=FACE_BOUND ( 'NONE', #99, .T. ) ;
#8208=CIRCLE ( 'NONE', #4447, 2.649999999999985700 ) ;
#8211=DIRECTION ( 'NONE',  ( 0.000000000000000000, 1.000000000000000000, 0.000000000000000000 ) ) ;
#8223=LINE ( 'NONE', #2306, #8161 ) ;
#8224=SHAPE_DEFINITION_REPRESENTATION ( #3996, #2707 ) ;
#8238=DIRECTION ( 'NONE',  ( -0.000000000000000000, 1.000000000000000000, -0.000000000000000000 ) ) ;
#8249=LINE ( 'NONE', #5057, #5306 ) ;
#8252=AXIS2_PLACEMENT_3D ( 'NONE', #2709, #5351, #8024 ) ;
#8257=AXIS2_PLACEMENT_3D ( 'NONE', #1292, #3958, #6596 ) ;
#8270=ORIENTED_EDGE ( 'NONE', *, *, #2407, .T. ) ;
#8280=CARTESIAN_POINT ( 'NONE',  ( -30.00000000000002842, -20.00000000000000000, 200.0000000000000000 ) ) ;
#8281=ORIENTED_EDGE ( 'NONE', *, *, #4284, .F. ) ;
#8285=FACE_BOUND ( 'NONE', #1325, .T. ) ;
#8286=ADVANCED_FACE ( 'NONE', ( #4135 ), #2914, .F. ) ;
#8304=ORIENTED_EDGE ( 'NONE', *, *, #3239, .F. ) ;
#8314=EDGE_CURVE ( 'NONE', #6891, #5441, #116, .T. ) ;
#8336=VECTOR ( 'NONE', #4967, 1000.000000000000000 ) ;
#8341=AXIS2_PLACEMENT_3D ( 'NONE', #2357, #996, #5196 ) ;
#8342=ORIENTED_EDGE ( 'NONE', *, *, #4844, .F. ) ;
#8349=EDGE_LOOP ( 'NONE', ( #6742, #3303 ) ) ;
#8354=ORIENTED_EDGE ( 'NONE', *, *, #1931, .T. ) ;
#8361=DIRECTION ( 'NONE',  ( 0.000000000000000000, 0.000000000000000000, 1.000000000000000000 ) ) ;
#8369=EDGE_CURVE ( 'NONE', #5141, #5928, #7135, .T. ) ;
#8379=FACE_OUTER_BOUND ( 'NONE', #3686, .T. ) ;
#8407=FACE_OUTER_BOUND ( 'NONE', #3090, .T. ) ;
#8411=FACE_OUTER_BOUND ( 'NONE', #811, .T. ) ;
#8433=EDGE_LOOP ( 'NONE', ( #1100, #4048, #1370, #3627 ) ) ;
#8436=EDGE_CURVE ( 'NONE', #1609, #6518, #3871, .T. ) ;
#8460=DIRECTION ( 'NONE',  ( 0.000000000000000000, 0.000000000000000000, 1.000000000000000000 ) ) ;
#8461=ORIENTED_EDGE ( 'NONE', *, *, #2493, .T. ) ;
#8473=DIRECTION ( 'NONE',  ( 0.000000000000000000, 0.000000000000000000, 1.000000000000000000 ) ) ;
#8475=CARTESIAN_POINT ( 'NONE',  ( 219.9999999999999716, -25.00000000000000000, 162.5000000000000853 ) ) ;
#8479=DIRECTION ( 'NONE',  ( 0.000000000000000000, 0.000000000000000000, 1.000000000000000000 ) ) ;
#8484=DIRECTION ( 'NONE',  ( 0.000000000000000000, 0.000000000000000000, 1.000000000000000000 ) ) ;
#8491=VERTEX_POINT ( 'NONE', #5287 ) ;
#8500=VERTEX_POINT ( 'NONE', #5246 ) ;
#8506=EDGE_CURVE ( 'NONE', #437, #8491, #34, .T. ) ;
#8514=ORIENTED_EDGE ( 'NONE', *, *, #1994, .F. ) ;
#8516=DIRECTION ( 'NONE',  ( 1.000000000000000000, 0.000000000000000000, -0.000000000000000000 ) ) ;
#8527=CIRCLE ( 'NONE', #1989, 2.649999999999985700 ) ;
#8553=CARTESIAN_POINT ( 'NONE',  ( 303.3333333333333144, -20.00000000000000000, 162.5000000000000853 ) ) ;
#8554=DIRECTION ( 'NONE',  ( 0.000000000000000000, 0.000000000000000000, 1.000000000000000000 ) ) ;
#8581=FACE_OUTER_BOUND ( 'NONE', #1031, .T. ) ;
#8584=CARTESIAN_POINT ( 'NONE',  ( 176.0000000000000000, -20.00000000000000000, -86.63142504031547730 ) ) ;
#8589=EDGE_CURVE ( 'NONE', #1611, #1823, #4859, .T. ) ;
#8637=COLOUR_RGB('Dark Blue',0.08,0.2,0.34);
#8638=FILL_AREA_STYLE_COLOUR('',#8637);
#8639=FILL_AREA_STYLE('',(#8638));
#8640=SURFACE_STYLE_FILL_AREA(#8639);
#8641=SURFACE_SIDE_STYLE('',(#8640));
#8642=SURFACE_STYLE_USAGE(.BOTH.,#8641);
#8643=PRESENTATION_STYLE_ASSIGNMENT((#8642));
ENDSEC;
END-ISO-10303-21;
